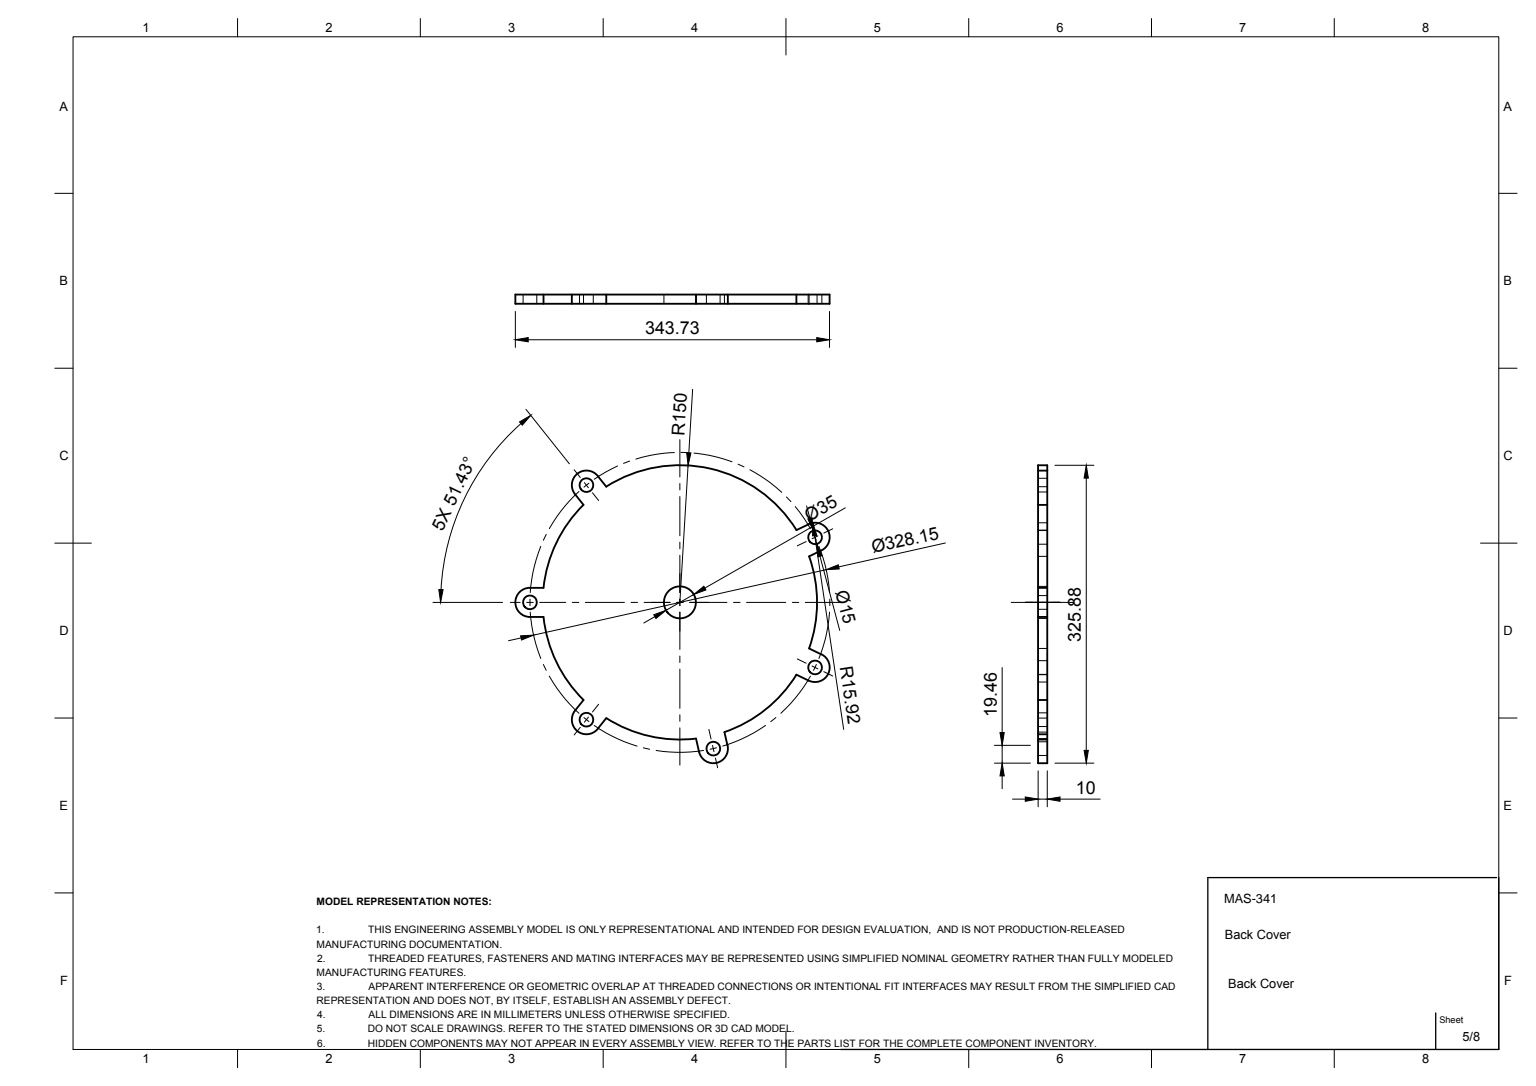
ISO-10303-21;
HEADER;
FILE_DESCRIPTION (('STEP AP214'),
    '1' );
FILE_NAME ('Back Cover.step',
    '2026-10-08T00:39:10',
    ( '' ),
    ( '' ),
    'SwSTEP 2.0',
    'SolidWorks 2025',
    '' );
FILE_SCHEMA (( 'AUTOMOTIVE_DESIGN' ));
ENDSEC;

DATA;
#4=PRODUCT ( 'Back Cover', 'Back Cover', '', ( #531 ) ) ;
#10=VERTEX_POINT ( 'NONE', #9173 ) ;
#12=( GEOMETRIC_REPRESENTATION_CONTEXT ( 3 ) GLOBAL_UNCERTAINTY_ASSIGNED_CONTEXT ( ( #1291 ) ) GLOBAL_UNIT_ASSIGNED_CONTEXT ( ( #18131, #16699, #13613 ) ) REPRESENTATION_CONTEXT ( 'NONE', 'WORKASPACE' ) );
#25=ORIENTED_EDGE ( 'NONE', *, *, #13470, .F. ) ;
#39=DIRECTION ( 'NONE',  ( 0.000000000000000000, 0.000000000000000000, 1.000000000000000000 ) ) ;
#57=CARTESIAN_POINT ( 'NONE',  ( -50.37374754117255549, -141.2886604036510221, 60.00000000000000000 ) ) ;
#62=ORIENTED_EDGE ( 'NONE', *, *, #6982, .T. ) ;
#74=DIRECTION ( 'NONE',  ( -0.000000000000000000, -0.000000000000000000, -1.000000000000000000 ) ) ;
#80=EDGE_LOOP ( 'NONE', ( #725, #12520, #18539, #7460 ) ) ;
#92=CARTESIAN_POINT ( 'NONE',  ( 128.2779226595531270, 102.2982297021113141, 60.00000000000000000 ) ) ;
#95=ORIENTED_EDGE ( 'NONE', *, *, #17125, .F. ) ;
#100=FACE_BOUND ( 'NONE', #8738, .T. ) ;
#107=SURFACE_SIDE_STYLE ('',( #15666 ) ) ;
#135=EDGE_CURVE ( 'NONE', #17975, #14483, #10909, .T. ) ;
#136=CARTESIAN_POINT ( 'NONE',  ( 141.8714406926368099, -48.70825716237082759, 49.99999999999999289 ) ) ;
#173=VECTOR ( 'NONE', #8479, 1000.000000000000000 ) ;
#176=FACE_BOUND ( 'NONE', #16626, .T. ) ;
#187=CYLINDRICAL_SURFACE ( 'NONE', #11980, 150.0000000000000284 ) ;
#205=ORIENTED_EDGE ( 'NONE', *, *, #13470, .T. ) ;
#208=DIRECTION ( 'NONE',  ( 1.000000000000000000, 0.000000000000000000, 0.000000000000000000 ) ) ;
#212=FACE_OUTER_BOUND ( 'NONE', #80, .T. ) ;
#232=DIRECTION ( 'NONE',  ( 1.000000000000000000, 0.000000000000000000, 0.000000000000000000 ) ) ;
#248=CIRCLE ( 'NONE', #6127, 15.91767397667354800 ) ;
#250=ORIENTED_EDGE ( 'NONE', *, *, #6281, .T. ) ;
#254=CARTESIAN_POINT ( 'NONE',  ( 15.91767397667354800, 164.0736214083062805, 49.99999999999999289 ) ) ;
#258=EDGE_CURVE ( 'NONE', #16031, #14304, #11946, .T. ) ;
#262=EDGE_CURVE ( 'NONE', #18721, #13125, #19565, .T. ) ;
#277=FACE_OUTER_BOUND ( 'NONE', #4264, .T. ) ;
#282=DIRECTION ( 'NONE',  ( 4.650550193362991910E-16, 1.000000000000000000, 0.000000000000000000 ) ) ;
#304=FACE_BOUND ( 'NONE', #20117, .T. ) ;
#328=CARTESIAN_POINT ( 'NONE',  ( 85.53020504959901871, -140.9188050298377846, 60.00000000000000000 ) ) ;
#344=VECTOR ( 'NONE', #11455, 1000.000000000000000 ) ;
#372=DIRECTION ( 'NONE',  ( -0.000000000000000000, -0.000000000000000000, -1.000000000000000000 ) ) ;
#377=CARTESIAN_POINT ( 'NONE',  ( 0.000000000000000000, 0.000000000000000000, 49.99999999999999289 ) ) ;
#389=DIRECTION ( 'NONE',  ( -1.000000000000000000, 0.000000000000000000, 0.000000000000000000 ) ) ;
#402=LINE ( 'NONE', #6654, #2889 ) ;
#403=DIRECTION ( 'NONE',  ( 1.000000000000000000, 0.000000000000000000, -0.000000000000000000 ) ) ;
#431=ORIENTED_EDGE ( 'NONE', *, *, #9079, .T. ) ;
#442=DIRECTION ( 'NONE',  ( -0.000000000000000000, -0.000000000000000000, -1.000000000000000000 ) ) ;
#473=VECTOR ( 'NONE', #13912, 1000.000000000000000 ) ;
#531=PRODUCT_CONTEXT ( 'NONE', #16261, 'mechanical' ) ;
#599=VERTEX_POINT ( 'NONE', #13287 ) ;
#600=FACE_OUTER_BOUND ( 'NONE', #14957, .T. ) ;
#615=FACE_OUTER_BOUND ( 'NONE', #9474, .T. ) ;
#625=VERTEX_POINT ( 'NONE', #8798 ) ;
#698=VERTEX_POINT ( 'NONE', #1222 ) ;
#706=ORIENTED_EDGE ( 'NONE', *, *, #12017, .T. ) ;
#711=ORIENTED_EDGE ( 'NONE', *, *, #14248, .F. ) ;
#718=DIRECTION ( 'NONE',  ( -0.9749279121818223981, -0.2225209339563194721, 0.000000000000000000 ) ) ;
#725=ORIENTED_EDGE ( 'NONE', *, *, #984, .T. ) ;
#741=CARTESIAN_POINT ( 'NONE',  ( 141.8714406926368099, -48.70825716237082759, 60.00000000000000000 ) ) ;
#743=CIRCLE ( 'NONE', #20010, 15.91767397667354089 ) ;
#760=CARTESIAN_POINT ( 'NONE',  ( 56.84754764479241373, -154.7316448359447634, 60.00000000000000000 ) ) ;
#773=LINE ( 'NONE', #10087, #5009 ) ;
#778=DIRECTION ( 'NONE',  ( 1.000000000000000000, 0.000000000000000000, 0.000000000000000000 ) ) ;
#798=CARTESIAN_POINT ( 'NONE',  ( 128.2779226595531270, 102.2982297021113141, 60.00000000000000000 ) ) ;
#813=ORIENTED_EDGE ( 'NONE', *, *, #1509, .F. ) ;
#833=AXIS2_PLACEMENT_3D ( 'NONE', #13835, #20185, #6186 ) ;
#847=ADVANCED_FACE ( 'NONE', ( #7869, #100, #5022, #11349, #3578, #17601, #304, #15753 ), #19234, .F. ) ;
#856=DIRECTION ( 'NONE',  ( -1.000000000000000000, 0.000000000000000000, 0.000000000000000000 ) ) ;
#882=DIRECTION ( 'NONE',  ( -0.000000000000000000, -0.000000000000000000, -1.000000000000000000 ) ) ;
#889=EDGE_LOOP ( 'NONE', ( #62, #9459, #3655, #15133 ) ) ;
#893=CIRCLE ( 'NONE', #19539, 15.91767397667354089 ) ;
#900=ORIENTED_EDGE ( 'NONE', *, *, #1584, .T. ) ;
#916=ORIENTED_EDGE ( 'NONE', *, *, #9093, .F. ) ;
#918=ORIENTED_EDGE ( 'NONE', *, *, #10465, .F. ) ;
#922=AXIS2_PLACEMENT_3D ( 'NONE', #2246, #13164, #10012 ) ;
#941=ORIENTED_EDGE ( 'NONE', *, *, #6979, .T. ) ;
#958=ORIENTED_EDGE ( 'NONE', *, *, #5414, .T. ) ;
#984=EDGE_CURVE ( 'NONE', #6115, #9946, #10014, .T. ) ;
#987=EDGE_CURVE ( 'NONE', #11007, #1319, #6991, .T. ) ;
#992=ORIENTED_EDGE ( 'NONE', *, *, #14786, .F. ) ;
#1011=CYLINDRICAL_SURFACE ( 'NONE', #6981, 17.50000000000000355 ) ;
#1018=FACE_OUTER_BOUND ( 'NONE', #6672, .T. ) ;
#1043=DIRECTION ( 'NONE',  ( -0.9749279121818226201, -0.2225209339563185285, 0.000000000000000000 ) ) ;
#1063=DIRECTION ( 'NONE',  ( 1.000000000000000000, 0.000000000000000000, 0.000000000000000000 ) ) ;
#1088=CARTESIAN_POINT ( 'NONE',  ( 71.18887634719571622, -147.8252249328912740, 60.00000000000000000 ) ) ;
#1092=CARTESIAN_POINT ( 'NONE',  ( 148.9554720520395392, -17.67108784863215476, 60.00000000000000000 ) ) ;
#1105=PLANE ( 'NONE',  #9572 ) ;
#1107=CARTESIAN_POINT ( 'NONE',  ( 71.18887634719571622, -147.8252249328912740, 60.00000000000000000 ) ) ;
#1113=( GEOMETRIC_REPRESENTATION_CONTEXT ( 3 ) GLOBAL_UNCERTAINTY_ASSIGNED_CONTEXT ( ( #10482 ) ) GLOBAL_UNIT_ASSIGNED_CONTEXT ( ( #20157, #10630, #1338 ) ) REPRESENTATION_CONTEXT ( 'NONE', 'WORKASPACE' ) );
#1133=ORIENTED_EDGE ( 'NONE', *, *, #5414, .F. ) ;
#1142=DIRECTION ( 'NONE',  ( 1.000000000000000000, 0.000000000000000000, 0.000000000000000000 ) ) ;
#1150=AXIS2_PLACEMENT_3D ( 'NONE', #10589, #13768, #9061 ) ;
#1174=CYLINDRICAL_SURFACE ( 'NONE', #13335, 7.500000000000020428 ) ;
#1181=AXIS2_PLACEMENT_3D ( 'NONE', #18694, #7526, #4675 ) ;
#1195=LINE ( 'NONE', #13780, #11300 ) ;
#1222=CARTESIAN_POINT ( 'NONE',  ( -150.0000000000000284, 0.000000000000000000, 60.00000000000000000 ) ) ;
#1247=AXIS2_PLACEMENT_3D ( 'NONE', #7167, #11750, #11657 ) ;
#1257=CARTESIAN_POINT ( 'NONE',  ( 141.8714406926368099, -48.70825716237082759, 60.00000000000000000 ) ) ;
#1289=DIRECTION ( 'NONE',  ( -0.000000000000000000, -0.000000000000000000, -1.000000000000000000 ) ) ;
#1291=UNCERTAINTY_MEASURE_WITH_UNIT (LENGTH_MEASURE( 1.000000000000000082E-05 ), #18131, 'distance_accuracy_value', 'NONE');
#1305=FACE_BOUND ( 'NONE', #15828, .T. ) ;
#1307=CYLINDRICAL_SURFACE ( 'NONE', #14633, 17.50000000000000355 ) ;
#1319=VERTEX_POINT ( 'NONE', #4241 ) ;
#1326=CARTESIAN_POINT ( 'NONE',  ( 0.000000000000000000, 164.0736214083062805, 60.00000000000000000 ) ) ;
#1338=( NAMED_UNIT ( * ) SI_UNIT ( $, .STERADIAN. ) SOLID_ANGLE_UNIT ( ) );
#1349=AXIS2_PLACEMENT_3D ( 'NONE', #5968, #6073, #13726 ) ;
#1353=VERTEX_POINT ( 'NONE', #2819 ) ;
#1363=LINE ( 'NONE', #10556, #11446 ) ;
#1364=FACE_OUTER_BOUND ( 'NONE', #20043, .T. ) ;
#1380=CARTESIAN_POINT ( 'NONE',  ( 118.3534152657848608, 114.7431683447366595, 60.00000000000000000 ) ) ;
#1381=ORIENTED_EDGE ( 'NONE', *, *, #135, .F. ) ;
#1385=ORIENTED_EDGE ( 'NONE', *, *, #16744, .T. ) ;
#1390=CIRCLE ( 'NONE', #8571, 150.0000000000000284 ) ;
#1400=AXIS2_PLACEMENT_3D ( 'NONE', #17477, #9487, #3450 ) ;
#1418=CIRCLE ( 'NONE', #15461, 150.0000000000000284 ) ;
#1445=DIRECTION ( 'NONE',  ( -0.000000000000000000, -0.000000000000000000, -1.000000000000000000 ) ) ;
#1472=EDGE_CURVE ( 'NONE', #8799, #13849, #8940, .T. ) ;
#1509=EDGE_CURVE ( 'NONE', #4476, #12253, #6504, .T. ) ;
#1519=LINE ( 'NONE', #7852, #19488 ) ;
#1524=CARTESIAN_POINT ( 'NONE',  ( 17.50000000000001776, 2.143131898507868643E-15, 60.00000000000000000 ) ) ;
#1529=AXIS2_PLACEMENT_3D ( 'NONE', #19924, #15537, #18818 ) ;
#1552=AXIS2_PLACEMENT_3D ( 'NONE', #4912, #17489, #14204 ) ;
#1579=AXIS2_PLACEMENT_3D ( 'NONE', #1380, #7217, #12522 ) ;
#1581=ORIENTED_EDGE ( 'NONE', *, *, #6806, .T. ) ;
#1584=EDGE_CURVE ( 'NONE', #11084, #12677, #9359, .T. ) ;
#1604=EDGE_LOOP ( 'NONE', ( #11796, #250, #431, #18706 ) ) ;
#1610=ORIENTED_EDGE ( 'NONE', *, *, #6423, .F. ) ;
#1617=DIRECTION ( 'NONE',  ( 1.000000000000000000, 0.000000000000000000, -0.000000000000000000 ) ) ;
#1632=CARTESIAN_POINT ( 'NONE',  ( 85.53020504959901871, -140.9188050298377846, 60.00000000000000000 ) ) ;
#1641=DIRECTION ( 'NONE',  ( -0.000000000000000000, -0.000000000000000000, -1.000000000000000000 ) ) ;
#1643=ADVANCED_BREP_SHAPE_REPRESENTATION ( '', ( #14854, #18639 ), #12 ) ;
#1668=ORIENTED_EDGE ( 'NONE', *, *, #10953, .T. ) ;
#1674=LINE ( 'NONE', #5228, #9676 ) ;
#1681=VERTEX_POINT ( 'NONE', #19287 ) ;
#1690=CARTESIAN_POINT ( 'NONE',  ( -152.4599531637108498, -36.50981547337168109, 60.00000000000000000 ) ) ;
#1697=DIRECTION ( 'NONE',  ( 1.000000000000000000, 0.000000000000000000, 0.000000000000000000 ) ) ;
#1711=CARTESIAN_POINT ( 'NONE',  ( 0.000000000000000000, 164.0736214083062805, 49.99999999999999289 ) ) ;
#1735=ORIENTED_EDGE ( 'NONE', *, *, #7341, .T. ) ;
#1740=EDGE_CURVE ( 'NONE', #6676, #16987, #17142, .T. ) ;
#1778=DIRECTION ( 'NONE',  ( 0.000000000000000000, 0.000000000000000000, 1.000000000000000000 ) ) ;
#1782=ADVANCED_FACE ( 'NONE', ( #12080 ), #4425, .T. ) ;
#1806=EDGE_LOOP ( 'NONE', ( #13482, #12155, #3837, #11415 ) ) ;
#1818=DIRECTION ( 'NONE',  ( 1.000000000000000000, -4.650550193362991910E-16, 0.000000000000000000 ) ) ;
#1822=CARTESIAN_POINT ( 'NONE',  ( -156.4179374840092862, -52.02840013024096066, 49.99999999999999289 ) ) ;
#1828=CIRCLE ( 'NONE', #15542, 7.500000000000007105 ) ;
#1843=LINE ( 'NONE', #8280, #16385 ) ;
#1850=EDGE_CURVE ( 'NONE', #9217, #15200, #9187, .T. ) ;
#1873=CYLINDRICAL_SURFACE ( 'NONE', #16470, 15.91767397667354089 ) ;
#1887=VERTEX_POINT ( 'NONE', #4317 ) ;
#1888=CIRCLE ( 'NONE', #17570, 15.91767397667354089 ) ;
#1890=EDGE_LOOP ( 'NONE', ( #916, #3438, #11512, #2174 ) ) ;
#1897=LINE ( 'NONE', #11196, #7566 ) ;
#1903=EDGE_CURVE ( 'NONE', #17877, #8041, #1843, .T. ) ;
#1907=EDGE_CURVE ( 'NONE', #16556, #4476, #3003, .T. ) ;
#1926=LINE ( 'NONE', #17482, #13030 ) ;
#1998=PLANE ( 'NONE',  #3865 ) ;
#2007=CIRCLE ( 'NONE', #16700, 7.500000000000008882 ) ;
#2015=ADVANCED_FACE ( 'NONE', ( #9948 ), #13293, .T. ) ;
#2032=CARTESIAN_POINT ( 'NONE',  ( 152.4599531637113330, -36.50981547336952104, 60.00000000000000000 ) ) ;
#2035=CARTESIAN_POINT ( 'NONE',  ( 152.4599531637113330, -36.50981547336952104, 60.00000000000000000 ) ) ;
#2037=CYLINDRICAL_SURFACE ( 'NONE', #2496, 7.500000000000008882 ) ;
#2058=DIRECTION ( 'NONE',  ( 1.000000000000000000, 0.000000000000000000, 0.000000000000000000 ) ) ;
#2066=EDGE_LOOP ( 'NONE', ( #20041, #7947, #14391, #7069 ) ) ;
#2073=VECTOR ( 'NONE', #9324, 1000.000000000000114 ) ;
#2075=ORIENTED_EDGE ( 'NONE', *, *, #3500, .F. ) ;
#2082=ORIENTED_EDGE ( 'NONE', *, *, #2486, .T. ) ;
#2109=VERTEX_POINT ( 'NONE', #15142 ) ;
#2110=ORIENTED_EDGE ( 'NONE', *, *, #18540, .T. ) ;
#2133=CYLINDRICAL_SURFACE ( 'NONE', #18006, 7.500000000000007105 ) ;
#2140=LINE ( 'NONE', #17790, #20045 ) ;
#2143=VECTOR ( 'NONE', #3874, 1000.000000000000000 ) ;
#2168=DIRECTION ( 'NONE',  ( -1.000000000000000000, 0.000000000000000000, 0.000000000000000000 ) ) ;
#2172=ADVANCED_FACE ( 'NONE', ( #8056 ), #2133, .F. ) ;
#2174=ORIENTED_EDGE ( 'NONE', *, *, #10355, .F. ) ;
#2177=ADVANCED_FACE ( 'NONE', ( #16047 ), #13058, .F. ) ;
#2206=CARTESIAN_POINT ( 'NONE',  ( -71.18887634719365565, -147.8252249328922687, 60.00000000000000000 ) ) ;
#2240=ORIENTED_EDGE ( 'NONE', *, *, #12488, .F. ) ;
#2245=ORIENTED_EDGE ( 'NONE', *, *, #15519, .T. ) ;
#2246=CARTESIAN_POINT ( 'NONE',  ( 126.5370453525553671, 80.55045718954892209, 60.00000000000000000 ) ) ;
#2257=CARTESIAN_POINT ( 'NONE',  ( 0.000000000000000000, 0.000000000000000000, 49.99999999999999289 ) ) ;
#2269=VERTEX_POINT ( 'NONE', #8950 ) ;
#2273=VECTOR ( 'NONE', #9693, 1000.000000000000000 ) ;
#2302=ADVANCED_FACE ( 'NONE', ( #11913 ), #19800, .T. ) ;
#2330=CARTESIAN_POINT ( 'NONE',  ( -148.9554720520392834, -17.67108784863415138, 60.00000000000000000 ) ) ;
#2335=ORIENTED_EDGE ( 'NONE', *, *, #16292, .F. ) ;
#2359=CARTESIAN_POINT ( 'NONE',  ( 128.2779226595531270, 102.2982297021113141, 49.99999999999999289 ) ) ;
#2362=VERTEX_POINT ( 'NONE', #16735 ) ;
#2367=VECTOR ( 'NONE', #7281, 1000.000000000000000 ) ;
#2405=DIRECTION ( 'NONE',  ( -0.000000000000000000, -0.000000000000000000, -1.000000000000000000 ) ) ;
#2422=ORIENTED_EDGE ( 'NONE', *, *, #19415, .T. ) ;
#2429=CARTESIAN_POINT ( 'NONE',  ( -175.8776271403844191, -36.50981547337168109, 60.00000000000000000 ) ) ;
#2445=DIRECTION ( 'NONE',  ( -0.000000000000000000, -0.000000000000000000, -1.000000000000000000 ) ) ;
#2486=EDGE_CURVE ( 'NONE', #1353, #1681, #14082, .T. ) ;
#2496=AXIS2_PLACEMENT_3D ( 'NONE', #11129, #17390, #3567 ) ;
#2525=EDGE_CURVE ( 'NONE', #10243, #10598, #19835, .T. ) ;
#2540=CIRCLE ( 'NONE', #3850, 150.0000000000000284 ) ;
#2550=CARTESIAN_POINT ( 'NONE',  ( -63.68887634719364144, -147.8252249328922687, 49.99999999999999289 ) ) ;
#2553=AXIS2_PLACEMENT_3D ( 'NONE', #8742, #16438, #11428 ) ;
#2606=CARTESIAN_POINT ( 'NONE',  ( 118.3534152657848608, 114.7431683447366595, 60.00000000000000000 ) ) ;
#2630=EDGE_CURVE ( 'NONE', #7170, #17394, #19295, .T. ) ;
#2660=FACE_OUTER_BOUND ( 'NONE', #2066, .T. ) ;
#2663=EDGE_LOOP ( 'NONE', ( #8353, #3788, #6370, #3707 ) ) ;
#2673=EDGE_CURVE ( 'NONE', #19329, #4234, #19485, .T. ) ;
#2680=ORIENTED_EDGE ( 'NONE', *, *, #4734, .T. ) ;
#2702=DIRECTION ( 'NONE',  ( -0.000000000000000000, -0.000000000000000000, -1.000000000000000000 ) ) ;
#2720=VERTEX_POINT ( 'NONE', #5377 ) ;
#2762=FACE_OUTER_BOUND ( 'NONE', #5149, .T. ) ;
#2769=ADVANCED_FACE ( 'NONE', ( #4030 ), #3930, .F. ) ;
#2771=EDGE_LOOP ( 'NONE', ( #13142, #16829 ) ) ;
#2799=DIRECTION ( 'NONE',  ( -0.000000000000000000, -0.000000000000000000, -1.000000000000000000 ) ) ;
#2819=CARTESIAN_POINT ( 'NONE',  ( 78.68887634719573043, -147.8252249328912740, 49.99999999999999289 ) ) ;
#2822=DIRECTION ( 'NONE',  ( 0.000000000000000000, 0.000000000000000000, 1.000000000000000000 ) ) ;
#2861=CARTESIAN_POINT ( 'NONE',  ( 159.9599531637113330, -36.50981547336952104, 49.99999999999999289 ) ) ;
#2874=ADVANCED_FACE ( 'NONE', ( #19877 ), #13943, .F. ) ;
#2889=VECTOR ( 'NONE', #11447, 1000.000000000000000 ) ;
#2909=CIRCLE ( 'NONE', #10735, 7.500000000000007105 ) ;
#2931=APPLICATION_CONTEXT ( 'automotive_design' ) ;
#2936=VECTOR ( 'NONE', #1641, 1000.000000000000000 ) ;
#2941=ORIENTED_EDGE ( 'NONE', *, *, #2525, .T. ) ;
#2965=ORIENTED_EDGE ( 'NONE', *, *, #17308, .F. ) ;
#2967=ORIENTED_EDGE ( 'NONE', *, *, #5286, .T. ) ;
#2975=EDGE_CURVE ( 'NONE', #16978, #16987, #10665, .T. ) ;
#2986=ORIENTED_EDGE ( 'NONE', *, *, #19843, .F. ) ;
#2988=CARTESIAN_POINT ( 'NONE',  ( -156.4179374840092862, -52.02840013024096066, 49.99999999999999289 ) ) ;
#3003=LINE ( 'NONE', #19237, #3320 ) ;
#3015=CIRCLE ( 'NONE', #18700, 7.500000000000007105 ) ;
#3025=PLANE ( 'NONE',  #1579 ) ;
#3101=LINE ( 'NONE', #15578, #9580 ) ;
#3124=DIRECTION ( 'NONE',  ( -0.000000000000000000, -0.000000000000000000, -1.000000000000000000 ) ) ;
#3135=DIRECTION ( 'NONE',  ( 1.000000000000000000, 0.000000000000000000, 0.000000000000000000 ) ) ;
#3146=AXIS2_PLACEMENT_3D ( 'NONE', #17379, #3352, #9591 ) ;
#3160=EDGE_LOOP ( 'NONE', ( #19301, #4729, #13376, #19732 ) ) ;
#3192=DIRECTION ( 'NONE',  ( 0.000000000000000000, 0.000000000000000000, 1.000000000000000000 ) ) ;
#3195=ORIENTED_EDGE ( 'NONE', *, *, #8308, .T. ) ;
#3223=VECTOR ( 'NONE', #74, 1000.000000000000000 ) ;
#3229=ADVANCED_FACE ( 'NONE', ( #16398 ), #15050, .T. ) ;
#3231=CARTESIAN_POINT ( 'NONE',  ( 120.7779226595530986, 102.2982297021113141, 60.00000000000000000 ) ) ;
#3233=DIRECTION ( 'NONE',  ( 0.000000000000000000, 0.000000000000000000, 1.000000000000000000 ) ) ;
#3243=ADVANCED_FACE ( 'NONE', ( #7276 ), #7083, .T. ) ;
#3264=DIRECTION ( 'NONE',  ( -0.000000000000000000, -0.000000000000000000, -1.000000000000000000 ) ) ;
#3267=FACE_OUTER_BOUND ( 'NONE', #1604, .T. ) ;
#3275=PRODUCT_DEFINITION ( 'UNKNOWN', '', #10143, #7010 ) ;
#3308=CIRCLE ( 'NONE', #19312, 150.0000000000000284 ) ;
#3316=CARTESIAN_POINT ( 'NONE',  ( 159.9599531637113330, -36.50981547336952104, 60.00000000000000000 ) ) ;
#3320=VECTOR ( 'NONE', #3679, 1000.000000000000000 ) ;
#3327=DIRECTION ( 'NONE',  ( -0.7818314824680222541, -0.6234898018587428092, 0.000000000000000000 ) ) ;
#3330=CARTESIAN_POINT ( 'NONE',  ( 71.18887634719571622, -147.8252249328912740, 60.00000000000000000 ) ) ;
#3341=EDGE_LOOP ( 'NONE', ( #9492, #4784, #5801, #2110, #12859, #14208, #1735, #19633, #12646, #958, #17042, #11082, #11220, #15387, #15418, #2422, #7191, #11685, #1581, #3959, #19178, #18458, #2245, #18129, #7799, #17297, #2967 ) ) ;
#3352=DIRECTION ( 'NONE',  ( 0.000000000000000000, 0.000000000000000000, 1.000000000000000000 ) ) ;
#3391=DIRECTION ( 'NONE',  ( 0.000000000000000000, 0.000000000000000000, 1.000000000000000000 ) ) ;
#3401=EDGE_CURVE ( 'NONE', #17191, #3695, #12037, .T. ) ;
#3407=VECTOR ( 'NONE', #8574, 1000.000000000000000 ) ;
#3438=ORIENTED_EDGE ( 'NONE', *, *, #3401, .T. ) ;
#3450=DIRECTION ( 'NONE',  ( -0.4338837391175549008, -0.9009688679024205893, 0.000000000000000000 ) ) ;
#3452=DIRECTION ( 'NONE',  ( 0.000000000000000000, 0.000000000000000000, 1.000000000000000000 ) ) ;
#3453=EDGE_LOOP ( 'NONE', ( #11712, #4339, #4209, #20136 ) ) ;
#3457=CARTESIAN_POINT ( 'NONE',  ( 0.000000000000000000, 164.0736214083062805, 60.00000000000000000 ) ) ;
#3458=LINE ( 'NONE', #2032, #2273 ) ;
#3490=AXIS2_PLACEMENT_3D ( 'NONE', #3457, #15736, #19021 ) ;
#3491=ORIENTED_EDGE ( 'NONE', *, *, #17032, .T. ) ;
#3493=DIRECTION ( 'NONE',  ( -1.000000000000000000, 4.650550193362991910E-16, 0.000000000000000000 ) ) ;
#3494=CARTESIAN_POINT ( 'NONE',  ( 50.37374754117451658, -141.2886604036503115, 49.99999999999999289 ) ) ;
#3500=EDGE_CURVE ( 'NONE', #4491, #18721, #7194, .T. ) ;
#3515=DIRECTION ( 'NONE',  ( 0.4338837391175662250, -0.9009688679024151492, 0.000000000000000000 ) ) ;
#3558=FACE_OUTER_BOUND ( 'NONE', #9060, .T. ) ;
#3567=DIRECTION ( 'NONE',  ( -1.000000000000000000, 0.000000000000000000, 0.000000000000000000 ) ) ;
#3568=VECTOR ( 'NONE', #3852, 1000.000000000000227 ) ;
#3569=CIRCLE ( 'NONE', #3896, 150.0000000000000284 ) ;
#3577=PLANE ( 'NONE',  #922 ) ;
#3578=FACE_BOUND ( 'NONE', #16226, .T. ) ;
#3595=DIRECTION ( 'NONE',  ( -4.650550193362991910E-16, -1.000000000000000000, 0.000000000000000000 ) ) ;
#3601=ORIENTED_EDGE ( 'NONE', *, *, #6285, .T. ) ;
#3606=CARTESIAN_POINT ( 'NONE',  ( -85.53020504959707182, -140.9188050298390067, 49.99999999999999289 ) ) ;
#3617=FACE_OUTER_BOUND ( 'NONE', #19792, .T. ) ;
#3620=VERTEX_POINT ( 'NONE', #14922 ) ;
#3639=AXIS2_PLACEMENT_3D ( 'NONE', #5062, #11284, #4960 ) ;
#3642=EDGE_LOOP ( 'NONE', ( #9938, #13927 ) ) ;
#3655=ORIENTED_EDGE ( 'NONE', *, *, #17655, .F. ) ;
#3672=ORIENTED_EDGE ( 'NONE', *, *, #18599, .F. ) ;
#3674=DIRECTION ( 'NONE',  ( 1.000000000000000000, 0.000000000000000000, 0.000000000000000000 ) ) ;
#3679=DIRECTION ( 'NONE',  ( -0.000000000000000000, -0.000000000000000000, -1.000000000000000000 ) ) ;
#3695=VERTEX_POINT ( 'NONE', #16669 ) ;
#3699=CIRCLE ( 'NONE', #14151, 7.500000000000020428 ) ;
#3700=VERTEX_POINT ( 'NONE', #15326 ) ;
#3702=ORIENTED_EDGE ( 'NONE', *, *, #4419, .T. ) ;
#3707=ORIENTED_EDGE ( 'NONE', *, *, #6423, .T. ) ;
#3723=DIRECTION ( 'NONE',  ( 0.000000000000000000, 0.000000000000000000, 1.000000000000000000 ) ) ;
#3732=DIRECTION ( 'NONE',  ( 0.7818314824680226982, 0.6234898018587423651, 0.000000000000000000 ) ) ;
#3738=COLOUR_RGB ( '', 0.66274510, 0.83137255, 0.94901961) ;
#3756=CARTESIAN_POINT ( 'NONE',  ( -167.4599531637108782, -36.50981547337168109, 60.00000000000000000 ) ) ;
#3760=DIRECTION ( 'NONE',  ( -0.000000000000000000, -0.000000000000000000, -1.000000000000000000 ) ) ;
#3764=CARTESIAN_POINT ( 'NONE',  ( -50.37374754117255549, -141.2886604036510221, 60.00000000000000000 ) ) ;
#3788=ORIENTED_EDGE ( 'NONE', *, *, #19393, .F. ) ;
#3797=ORIENTED_EDGE ( 'NONE', *, *, #4544, .F. ) ;
#3837=ORIENTED_EDGE ( 'NONE', *, *, #10862, .T. ) ;
#3850=AXIS2_PLACEMENT_3D ( 'NONE', #12740, #19000, #17466 ) ;
#3852=DIRECTION ( 'NONE',  ( -0.9749279121818223981, -0.2225209339563194721, 0.000000000000000000 ) ) ;
#3855=EDGE_CURVE ( 'NONE', #4788, #2109, #15644, .T. ) ;
#3858=CARTESIAN_POINT ( 'NONE',  ( 135.7779226595531270, 102.2982297021113141, 49.99999999999999289 ) ) ;
#3859=LINE ( 'NONE', #8464, #5451 ) ;
#3865=AXIS2_PLACEMENT_3D ( 'NONE', #18551, #4426, #1043 ) ;
#3869=ORIENTED_EDGE ( 'NONE', *, *, #5675, .F. ) ;
#3874=DIRECTION ( 'NONE',  ( -0.000000000000000000, -0.000000000000000000, -1.000000000000000000 ) ) ;
#3880=CARTESIAN_POINT ( 'NONE',  ( -79.05640494597940915, -127.4758205975444270, 60.00000000000000000 ) ) ;
#3896=AXIS2_PLACEMENT_3D ( 'NONE', #11016, #14092, #15733 ) ;
#3897=EDGE_CURVE ( 'NONE', #16737, #6676, #19883, .T. ) ;
#3906=CARTESIAN_POINT ( 'NONE',  ( 50.37374754117451658, -141.2886604036503115, 60.00000000000000000 ) ) ;
#3911=ORIENTED_EDGE ( 'NONE', *, *, #5282, .T. ) ;
#3930=PLANE ( 'NONE',  #4819 ) ;
#3934=VERTEX_POINT ( 'NONE', #19222 ) ;
#3938=VERTEX_POINT ( 'NONE', #3858 ) ;
#3949=LINE ( 'NONE', #16446, #13934 ) ;
#3959=ORIENTED_EDGE ( 'NONE', *, *, #5121, .T. ) ;
#3967=FACE_OUTER_BOUND ( 'NONE', #15282, .T. ) ;
#3973=DIRECTION ( 'NONE',  ( 1.000000000000000000, 0.000000000000000000, 0.000000000000000000 ) ) ;
#3983=ORIENTED_EDGE ( 'NONE', *, *, #12666, .T. ) ;
#3996=AXIS2_PLACEMENT_3D ( 'NONE', #19556, #11767, #8709 ) ;
#4014=ORIENTED_EDGE ( 'NONE', *, *, #17032, .F. ) ;
#4030=FACE_OUTER_BOUND ( 'NONE', #13227, .T. ) ;
#4056=ORIENTED_EDGE ( 'NONE', *, *, #17125, .T. ) ;
#4064=DIRECTION ( 'NONE',  ( 1.000000000000000000, 0.000000000000000000, 0.000000000000000000 ) ) ;
#4069=ORIENTED_EDGE ( 'NONE', *, *, #5286, .F. ) ;
#4071=DIRECTION ( 'NONE',  ( 0.000000000000000000, 0.000000000000000000, 1.000000000000000000 ) ) ;
#4082=DIRECTION ( 'NONE',  ( 0.000000000000000000, 0.000000000000000000, 1.000000000000000000 ) ) ;
#4092=DIRECTION ( 'NONE',  ( -0.000000000000000000, -0.000000000000000000, -1.000000000000000000 ) ) ;
#4098=DIRECTION ( 'NONE',  ( 1.000000000000000000, 0.000000000000000000, 0.000000000000000000 ) ) ;
#4122=ORIENTED_EDGE ( 'NONE', *, *, #5532, .T. ) ;
#4129=DIRECTION ( 'NONE',  ( 0.000000000000000000, 0.000000000000000000, 1.000000000000000000 ) ) ;
#4166=VECTOR ( 'NONE', #10347, 1000.000000000000000 ) ;
#4183=AXIS2_PLACEMENT_3D ( 'NONE', #16892, #9107, #208 ) ;
#4191=CARTESIAN_POINT ( 'NONE',  ( -79.05640494597940915, -127.4758205975444270, 49.99999999999999289 ) ) ;
#4203=CYLINDRICAL_SURFACE ( 'NONE', #18192, 150.0000000000000284 ) ;
#4209=ORIENTED_EDGE ( 'NONE', *, *, #11907, .F. ) ;
#4234=VERTEX_POINT ( 'NONE', #9956 ) ;
#4235=CARTESIAN_POINT ( 'NONE',  ( -78.68887634719368407, -147.8252249328922687, 60.00000000000000000 ) ) ;
#4241=CARTESIAN_POINT ( 'NONE',  ( 135.7779226595531270, 102.2982297021113141, 60.00000000000000000 ) ) ;
#4247=EDGE_CURVE ( 'NONE', #1319, #3938, #19560, .T. ) ;
#4264=EDGE_LOOP ( 'NONE', ( #4368, #6719, #5070, #9063 ) ) ;
#4274=ORIENTED_EDGE ( 'NONE', *, *, #11719, .T. ) ;
#4283=CIRCLE ( 'NONE', #14745, 7.500000000000020428 ) ;
#4300=PRESENTATION_STYLE_ASSIGNMENT (( #7468 ) ) ;
#4317=CARTESIAN_POINT ( 'NONE',  ( -79.05640494597940915, -127.4758205975444270, 60.00000000000000000 ) ) ;
#4328=DIRECTION ( 'NONE',  ( 0.4338837391175509040, 0.9009688679024224767, 0.000000000000000000 ) ) ;
#4339=ORIENTED_EDGE ( 'NONE', *, *, #3855, .F. ) ;
#4367=ORIENTED_EDGE ( 'NONE', *, *, #1903, .T. ) ;
#4368=ORIENTED_EDGE ( 'NONE', *, *, #12488, .T. ) ;
#4371=CARTESIAN_POINT ( 'NONE',  ( 106.6880305650188347, 105.4403344747995988, 49.99999999999999289 ) ) ;
#4373=DIRECTION ( 'NONE',  ( 4.650550193362991910E-16, 1.000000000000000000, 0.000000000000000000 ) ) ;
#4374=CARTESIAN_POINT ( 'NONE',  ( -141.8714406926361562, -48.70825716237266079, 49.99999999999999289 ) ) ;
#4395=ORIENTED_EDGE ( 'NONE', *, *, #6979, .F. ) ;
#4419=EDGE_CURVE ( 'NONE', #18721, #17815, #6063, .T. ) ;
#4425=CYLINDRICAL_SURFACE ( 'NONE', #10923, 150.0000000000000284 ) ;
#4426=DIRECTION ( 'NONE',  ( -0.2225209339563185562, 0.9749279121818227312, 0.000000000000000000 ) ) ;
#4431=DIRECTION ( 'NONE',  ( -0.9749279121818255067, 0.2225209339563057331, 0.000000000000000000 ) ) ;
#4444=AXIS2_PLACEMENT_3D ( 'NONE', #10484, #15616, #18279 ) ;
#4463=CARTESIAN_POINT ( 'NONE',  ( -15.91767397667354800, 164.0736214083062805, 60.00000000000000000 ) ) ;
#4470=FACE_BOUND ( 'NONE', #2771, .T. ) ;
#4476=VERTEX_POINT ( 'NONE', #9008 ) ;
#4490=CYLINDRICAL_SURFACE ( 'NONE', #5988, 7.500000000000007105 ) ;
#4491=VERTEX_POINT ( 'NONE', #4622 ) ;
#4515=LINE ( 'NONE', #5853, #2073 ) ;
#4523=CIRCLE ( 'NONE', #17944, 17.50000000000000355 ) ;
#4544=EDGE_CURVE ( 'NONE', #1887, #17975, #4515, .T. ) ;
#4597=ORIENTED_EDGE ( 'NONE', *, *, #15010, .T. ) ;
#4606=ORIENTED_EDGE ( 'NONE', *, *, #1907, .T. ) ;
#4610=AXIS2_PLACEMENT_3D ( 'NONE', #3316, #11075, #19076 ) ;
#4615=LINE ( 'NONE', #9717, #8243 ) ;
#4619=EDGE_LOOP ( 'NONE', ( #19256, #12856, #8644, #12571 ) ) ;
#4622=CARTESIAN_POINT ( 'NONE',  ( -175.8776271403844191, -36.50981547337168109, 60.00000000000000000 ) ) ;
#4629=VERTEX_POINT ( 'NONE', #3494 ) ;
#4646=DIRECTION ( 'NONE',  ( 0.9009688679024225877, -0.4338837391175509595, 0.000000000000000000 ) ) ;
#4659=CARTESIAN_POINT ( 'NONE',  ( 118.3534152657848608, 114.7431683447366595, 49.99999999999999289 ) ) ;
#4666=ORIENTED_EDGE ( 'NONE', *, *, #6197, .F. ) ;
#4675=DIRECTION ( 'NONE',  ( 1.000000000000000000, 0.000000000000000000, 0.000000000000000000 ) ) ;
#4692=DIRECTION ( 'NONE',  ( -0.9009688679024161484, -0.4338837391175643932, 0.000000000000000000 ) ) ;
#4729=ORIENTED_EDGE ( 'NONE', *, *, #7736, .F. ) ;
#4733=ORIENTED_EDGE ( 'NONE', *, *, #18231, .T. ) ;
#4734=EDGE_CURVE ( 'NONE', #8237, #4476, #743, .T. ) ;
#4739=AXIS2_PLACEMENT_3D ( 'NONE', #18707, #4692, #10915 ) ;
#4744=AXIS2_PLACEMENT_3D ( 'NONE', #9033, #4129, #16145 ) ;
#4749=ADVANCED_FACE ( 'NONE', ( #19636 ), #1011, .F. ) ;
#4776=ADVANCED_FACE ( 'NONE', ( #2762 ), #4490, .F. ) ;
#4777=ORIENTED_EDGE ( 'NONE', *, *, #4870, .F. ) ;
#4784=ORIENTED_EDGE ( 'NONE', *, *, #9415, .T. ) ;
#4788=VERTEX_POINT ( 'NONE', #15437 ) ;
#4811=EDGE_LOOP ( 'NONE', ( #16003, #8956, #15930, #10927 ) ) ;
#4819=AXIS2_PLACEMENT_3D ( 'NONE', #10172, #16521, #14872 ) ;
#4827=DIRECTION ( 'NONE',  ( -0.000000000000000000, -0.000000000000000000, -1.000000000000000000 ) ) ;
#4855=CARTESIAN_POINT ( 'NONE',  ( 0.000000000000000000, 164.0736214083062805, 60.00000000000000000 ) ) ;
#4870=EDGE_CURVE ( 'NONE', #5317, #13849, #11547, .T. ) ;
#4877=DIRECTION ( 'NONE',  ( -1.000000000000000000, 0.000000000000000000, 0.000000000000000000 ) ) ;
#4888=ORIENTED_EDGE ( 'NONE', *, *, #19843, .T. ) ;
#4901=DIRECTION ( 'NONE',  ( 1.000000000000000000, 0.000000000000000000, 0.000000000000000000 ) ) ;
#4912=CARTESIAN_POINT ( 'NONE',  ( 159.9599531637113330, -36.50981547336952104, 60.00000000000000000 ) ) ;
#4926=CARTESIAN_POINT ( 'NONE',  ( 0.000000000000000000, 0.000000000000000000, 49.99999999999999289 ) ) ;
#4934=ORIENTED_EDGE ( 'NONE', *, *, #10382, .F. ) ;
#4940=EDGE_LOOP ( 'NONE', ( #18354, #4934, #19786, #15681 ) ) ;
#4955=ADVANCED_FACE ( 'NONE', ( #10928 ), #18826, .F. ) ;
#4960=DIRECTION ( 'NONE',  ( 1.000000000000000000, 0.000000000000000000, 0.000000000000000000 ) ) ;
#4964=AXIS2_PLACEMENT_3D ( 'NONE', #6977, #16300, #13196 ) ;
#4980=ORIENTED_EDGE ( 'NONE', *, *, #9415, .F. ) ;
#5000=DIRECTION ( 'NONE',  ( -0.000000000000000000, -0.000000000000000000, -1.000000000000000000 ) ) ;
#5005=DIRECTION ( 'NONE',  ( -1.000000000000000000, 0.000000000000000000, 0.000000000000000000 ) ) ;
#5008=VECTOR ( 'NONE', #18332, 1000.000000000000000 ) ;
#5009=VECTOR ( 'NONE', #19865, 1000.000000000000000 ) ;
#5015=DIRECTION ( 'NONE',  ( -1.000000000000000000, 0.000000000000000000, 0.000000000000000000 ) ) ;
#5022=FACE_BOUND ( 'NONE', #13984, .T. ) ;
#5025=VECTOR ( 'NONE', #15688, 1000.000000000000227 ) ;
#5030=DIRECTION ( 'NONE',  ( 0.000000000000000000, 0.000000000000000000, 1.000000000000000000 ) ) ;
#5062=CARTESIAN_POINT ( 'NONE',  ( -159.9599531637108782, -36.50981547337168109, 60.00000000000000000 ) ) ;
#5065=ORIENTED_EDGE ( 'NONE', *, *, #135, .T. ) ;
#5070=ORIENTED_EDGE ( 'NONE', *, *, #13129, .F. ) ;
#5083=VERTEX_POINT ( 'NONE', #19425 ) ;
#5121=EDGE_CURVE ( 'NONE', #10879, #7170, #1418, .T. ) ;
#5149=EDGE_LOOP ( 'NONE', ( #19102, #15112, #4777, #11521 ) ) ;
#5163=DIRECTION ( 'NONE',  ( -0.000000000000000000, -0.000000000000000000, -1.000000000000000000 ) ) ;
#5181=DIRECTION ( 'NONE',  ( -0.9749279121818255067, 0.2225209339563057331, 0.000000000000000000 ) ) ;
#5196=DIRECTION ( 'NONE',  ( 1.000000000000000000, 0.000000000000000000, 0.000000000000000000 ) ) ;
#5197=CIRCLE ( 'NONE', #14001, 15.91767397667354089 ) ;
#5203=ORIENTED_EDGE ( 'NONE', *, *, #18109, .F. ) ;
#5204=DIRECTION ( 'NONE',  ( 0.2225209339563194721, -0.9749279121818225091, 0.000000000000000000 ) ) ;
#5209=DIRECTION ( 'NONE',  ( -0.000000000000000000, -0.000000000000000000, -1.000000000000000000 ) ) ;
#5223=CARTESIAN_POINT ( 'NONE',  ( 17.50000000000001776, 2.143131898507868643E-15, 60.00000000000000000 ) ) ;
#5228=CARTESIAN_POINT ( 'NONE',  ( -15.91767397667354800, 164.0736214083062805, 60.00000000000000000 ) ) ;
#5251=EDGE_CURVE ( 'NONE', #12873, #10598, #2140, .T. ) ;
#5281=EDGE_LOOP ( 'NONE', ( #14805, #992, #6577, #17055 ) ) ;
#5282=EDGE_CURVE ( 'NONE', #5083, #3700, #7694, .T. ) ;
#5286=EDGE_CURVE ( 'NONE', #3620, #16612, #8955, .T. ) ;
#5288=ORIENTED_EDGE ( 'NONE', *, *, #9531, .F. ) ;
#5300=DIRECTION ( 'NONE',  ( 1.000000000000000000, 0.000000000000000000, 0.000000000000000000 ) ) ;
#5316=CARTESIAN_POINT ( 'NONE',  ( -7.500000000000008882, 164.0736214083062805, 60.00000000000000000 ) ) ;
#5317=VERTEX_POINT ( 'NONE', #10695 ) ;
#5323=DIRECTION ( 'NONE',  ( -0.000000000000000000, -0.000000000000000000, -1.000000000000000000 ) ) ;
#5377=CARTESIAN_POINT ( 'NONE',  ( -56.84754764479025368, -154.7316448359455308, 60.00000000000000000 ) ) ;
#5382=CIRCLE ( 'NONE', #7322, 15.91767397667354089 ) ;
#5391=AXIS2_PLACEMENT_3D ( 'NONE', #19017, #1818, #282 ) ;
#5400=DIRECTION ( 'NONE',  ( -0.000000000000000000, -0.000000000000000000, -1.000000000000000000 ) ) ;
#5406=DIRECTION ( 'NONE',  ( 0.000000000000000000, 0.000000000000000000, 1.000000000000000000 ) ) ;
#5408=ORIENTED_EDGE ( 'NONE', *, *, #10832, .F. ) ;
#5414=EDGE_CURVE ( 'NONE', #6230, #2720, #5749, .T. ) ;
#5416=LINE ( 'NONE', #5223, #2143 ) ;
#5425=ORIENTED_EDGE ( 'NONE', *, *, #12017, .F. ) ;
#5446=DIRECTION ( 'NONE',  ( -0.000000000000000000, -0.000000000000000000, -1.000000000000000000 ) ) ;
#5451=VECTOR ( 'NONE', #882, 1000.000000000000000 ) ;
#5452=CARTESIAN_POINT ( 'NONE',  ( 126.5370453525553671, 80.55045718954892209, 49.99999999999999289 ) ) ;
#5471=VECTOR ( 'NONE', #16136, 1000.000000000000227 ) ;
#5479=ADVANCED_FACE ( 'NONE', ( #1364 ), #7593, .T. ) ;
#5498=EDGE_LOOP ( 'NONE', ( #4980, #14689, #7232, #6679 ) ) ;
#5519=DIRECTION ( 'NONE',  ( 0.000000000000000000, 0.000000000000000000, 1.000000000000000000 ) ) ;
#5532=EDGE_CURVE ( 'NONE', #16978, #16737, #12264, .T. ) ;
#5557=CARTESIAN_POINT ( 'NONE',  ( -156.4179374840092862, -52.02840013024096066, 60.00000000000000000 ) ) ;
#5576=EDGE_LOOP ( 'NONE', ( #7626, #17569, #4274, #4395 ) ) ;
#5581=FACE_OUTER_BOUND ( 'NONE', #14740, .T. ) ;
#5590=FACE_OUTER_BOUND ( 'NONE', #5576, .T. ) ;
#5593=CARTESIAN_POINT ( 'NONE',  ( 128.2779226595531270, 102.2982297021113141, 60.00000000000000000 ) ) ;
#5625=DIRECTION ( 'NONE',  ( -0.000000000000000000, -0.000000000000000000, -1.000000000000000000 ) ) ;
#5639=AXIS2_PLACEMENT_3D ( 'NONE', #7350, #10218, #19445 ) ;
#5645=CARTESIAN_POINT ( 'NONE',  ( 0.000000000000000000, 0.000000000000000000, 60.00000000000000000 ) ) ;
#5661=DIRECTION ( 'NONE',  ( -0.000000000000000000, -0.000000000000000000, -1.000000000000000000 ) ) ;
#5675=EDGE_CURVE ( 'NONE', #4234, #2109, #20125, .T. ) ;
#5681=EDGE_LOOP ( 'NONE', ( #5425, #11818, #5065, #4733 ) ) ;
#5708=DIRECTION ( 'NONE',  ( 0.000000000000000000, 0.000000000000000000, 1.000000000000000000 ) ) ;
#5719=DIRECTION ( 'NONE',  ( -1.000000000000000000, 0.000000000000000000, 0.000000000000000000 ) ) ;
#5731=CYLINDRICAL_SURFACE ( 'NONE', #14969, 15.91767397667354800 ) ;
#5749=CIRCLE ( 'NONE', #16211, 15.91767397667354089 ) ;
#5776=ORIENTED_EDGE ( 'NONE', *, *, #1850, .F. ) ;
#5790=EDGE_LOOP ( 'NONE', ( #8970, #8483, #14543, #4606 ) ) ;
#5795=CARTESIAN_POINT ( 'NONE',  ( 78.68887634719573043, -147.8252249328912740, 60.00000000000000000 ) ) ;
#5796=FACE_OUTER_BOUND ( 'NONE', #16439, .T. ) ;
#5801=ORIENTED_EDGE ( 'NONE', *, *, #10832, .T. ) ;
#5818=CARTESIAN_POINT ( 'NONE',  ( 0.000000000000000000, 164.0736214083062805, 60.00000000000000000 ) ) ;
#5821=CARTESIAN_POINT ( 'NONE',  ( 0.000000000000000000, 164.0736214083062805, 49.99999999999999289 ) ) ;
#5823=CARTESIAN_POINT ( 'NONE',  ( 79.05640494598117129, -127.4758205975433327, 49.99999999999999289 ) ) ;
#5853=CARTESIAN_POINT ( 'NONE',  ( -79.05640494597940915, -127.4758205975444270, 60.00000000000000000 ) ) ;
#5856=VECTOR ( 'NONE', #14308, 1000.000000000000227 ) ;
#5908=ORIENTED_EDGE ( 'NONE', *, *, #2975, .F. ) ;
#5918=AXIS2_PLACEMENT_3D ( 'NONE', #7723, #13963, #3135 ) ;
#5968=CARTESIAN_POINT ( 'NONE',  ( 0.000000000000000000, 0.000000000000000000, 49.99999999999999289 ) ) ;
#5987=EDGE_CURVE ( 'NONE', #3620, #6087, #1674, .T. ) ;
#5988=AXIS2_PLACEMENT_3D ( 'NONE', #12458, #12360, #15545 ) ;
#6032=VECTOR ( 'NONE', #14986, 1000.000000000000000 ) ;
#6037=DIRECTION ( 'NONE',  ( -1.000000000000000000, 0.000000000000000000, 0.000000000000000000 ) ) ;
#6063=LINE ( 'NONE', #12068, #5008 ) ;
#6068=ORIENTED_EDGE ( 'NONE', *, *, #18801, .T. ) ;
#6073=DIRECTION ( 'NONE',  ( 0.000000000000000000, 0.000000000000000000, 1.000000000000000000 ) ) ;
#6083=CARTESIAN_POINT ( 'NONE',  ( -63.68887634719364144, -147.8252249328922687, 60.00000000000000000 ) ) ;
#6087=VERTEX_POINT ( 'NONE', #10967 ) ;
#6090=VECTOR ( 'NONE', #13617, 1000.000000000000227 ) ;
#6115=VERTEX_POINT ( 'NONE', #13170 ) ;
#6125=CARTESIAN_POINT ( 'NONE',  ( -150.0000000000000284, 0.000000000000000000, 60.00000000000000000 ) ) ;
#6127=AXIS2_PLACEMENT_3D ( 'NONE', #5821, #13577, #12042 ) ;
#6129=CARTESIAN_POINT ( 'NONE',  ( -87.10655032386719654, -147.8252249328922687, 60.00000000000000000 ) ) ;
#6144=VECTOR ( 'NONE', #19755, 1000.000000000000114 ) ;
#6153=CIRCLE ( 'NONE', #10060, 7.500000000000008882 ) ;
#6186=DIRECTION ( 'NONE',  ( -1.000000000000000000, 0.000000000000000000, 0.000000000000000000 ) ) ;
#6197=EDGE_CURVE ( 'NONE', #9011, #14411, #8776, .T. ) ;
#6230=VERTEX_POINT ( 'NONE', #6129 ) ;
#6251=CARTESIAN_POINT ( 'NONE',  ( -148.9554720520392834, -17.67108784863415138, 60.00000000000000000 ) ) ;
#6281=EDGE_CURVE ( 'NONE', #6717, #12028, #9019, .T. ) ;
#6285=EDGE_CURVE ( 'NONE', #17700, #8237, #1519, .T. ) ;
#6290=LINE ( 'NONE', #136, #8230 ) ;
#6301=ADVANCED_FACE ( 'NONE', ( #17484 ), #8054, .F. ) ;
#6320=CIRCLE ( 'NONE', #17749, 150.0000000000000284 ) ;
#6341=CARTESIAN_POINT ( 'NONE',  ( -15.91767397667354800, 164.0736214083062805, 49.99999999999999289 ) ) ;
#6367=CARTESIAN_POINT ( 'NONE',  ( -85.53020504959707182, -140.9188050298390067, 60.00000000000000000 ) ) ;
#6369=ADVANCED_FACE ( 'NONE', ( #11526 ), #12956, .F. ) ;
#6370=ORIENTED_EDGE ( 'NONE', *, *, #7341, .F. ) ;
#6423=EDGE_CURVE ( 'NONE', #13125, #9217, #3949, .T. ) ;
#6429=DIRECTION ( 'NONE',  ( 0.000000000000000000, 0.000000000000000000, 1.000000000000000000 ) ) ;
#6432=ORIENTED_EDGE ( 'NONE', *, *, #16130, .T. ) ;
#6434=DIRECTION ( 'NONE',  ( -0.000000000000000000, -0.000000000000000000, -1.000000000000000000 ) ) ;
#6442=CARTESIAN_POINT ( 'NONE',  ( 0.000000000000000000, 0.000000000000000000, 60.00000000000000000 ) ) ;
#6462=VERTEX_POINT ( 'NONE', #5795 ) ;
#6504=LINE ( 'NONE', #4659, #9941 ) ;
#6557=DIRECTION ( 'NONE',  ( 0.000000000000000000, 0.000000000000000000, 1.000000000000000000 ) ) ;
#6569=LINE ( 'NONE', #10946, #11966 ) ;
#6571=CIRCLE ( 'NONE', #7863, 150.0000000000000284 ) ;
#6572=CARTESIAN_POINT ( 'NONE',  ( 0.000000000000000000, 0.000000000000000000, 60.00000000000000000 ) ) ;
#6577=ORIENTED_EDGE ( 'NONE', *, *, #15894, .F. ) ;
#6615=DIRECTION ( 'NONE',  ( 0.000000000000000000, 0.000000000000000000, 1.000000000000000000 ) ) ;
#6631=ORIENTED_EDGE ( 'NONE', *, *, #5121, .F. ) ;
#6654=CARTESIAN_POINT ( 'NONE',  ( 120.7779226595530986, 102.2982297021113141, 60.00000000000000000 ) ) ;
#6672=EDGE_LOOP ( 'NONE', ( #4056, #14230, #918, #12943 ) ) ;
#6676=VERTEX_POINT ( 'NONE', #9364 ) ;
#6679=ORIENTED_EDGE ( 'NONE', *, *, #11610, .F. ) ;
#6700=VERTEX_POINT ( 'NONE', #57 ) ;
#6717=VERTEX_POINT ( 'NONE', #10478 ) ;
#6719=ORIENTED_EDGE ( 'NONE', *, *, #13494, .F. ) ;
#6728=PLANE ( 'NONE',  #5391 ) ;
#6742=VECTOR ( 'NONE', #4373, 1000.000000000000000 ) ;
#6750=CARTESIAN_POINT ( 'NONE',  ( 7.500000000000008882, 164.0736214083062805, 49.99999999999999289 ) ) ;
#6767=AXIS2_PLACEMENT_3D ( 'NONE', #12658, #5204, #18920 ) ;
#6770=CARTESIAN_POINT ( 'NONE',  ( 15.91767397667354089, 149.1530343478547422, 60.00000000000000000 ) ) ;
#6777=ORIENTED_EDGE ( 'NONE', *, *, #5251, .T. ) ;
#6806=EDGE_CURVE ( 'NONE', #11084, #10879, #1897, .T. ) ;
#6820=CIRCLE ( 'NONE', #15335, 15.91767397667355510 ) ;
#6942=LINE ( 'NONE', #3764, #9908 ) ;
#6943=ORIENTED_EDGE ( 'NONE', *, *, #17547, .F. ) ;
#6955=DIRECTION ( 'NONE',  ( -0.000000000000000000, -0.000000000000000000, -1.000000000000000000 ) ) ;
#6959=CYLINDRICAL_SURFACE ( 'NONE', #5639, 15.91767397667354089 ) ;
#6977=CARTESIAN_POINT ( 'NONE',  ( 0.000000000000000000, 0.000000000000000000, 60.00000000000000000 ) ) ;
#6979=EDGE_CURVE ( 'NONE', #3938, #16337, #3015, .T. ) ;
#6981=AXIS2_PLACEMENT_3D ( 'NONE', #11564, #5625, #2168 ) ;
#6982=EDGE_CURVE ( 'NONE', #14304, #8041, #6290, .T. ) ;
#6991=CIRCLE ( 'NONE', #16785, 7.500000000000007105 ) ;
#7010=PRODUCT_DEFINITION_CONTEXT ( 'detailed design', #2931, 'design' ) ;
#7060=CARTESIAN_POINT ( 'NONE',  ( -63.68887634719364144, -147.8252249328922687, 60.00000000000000000 ) ) ;
#7069=ORIENTED_EDGE ( 'NONE', *, *, #2486, .F. ) ;
#7083=CYLINDRICAL_SURFACE ( 'NONE', #3996, 15.91767397667354800 ) ;
#7091=SHAPE_REPRESENTATION_RELATIONSHIP ( 'NONE' , 'NONE' ,  #7558, #1643 ) ;
#7098=DIRECTION ( 'NONE',  ( 1.000000000000000000, 0.000000000000000000, 0.000000000000000000 ) ) ;
#7117=VERTEX_POINT ( 'NONE', #11675 ) ;
#7157=VECTOR ( 'NONE', #6434, 1000.000000000000000 ) ;
#7167=CARTESIAN_POINT ( 'NONE',  ( -71.18887634719365565, -147.8252249328922687, 60.00000000000000000 ) ) ;
#7170=VERTEX_POINT ( 'NONE', #17732 ) ;
#7181=EDGE_CURVE ( 'NONE', #13002, #1681, #19463, .T. ) ;
#7190=CARTESIAN_POINT ( 'NONE',  ( 135.7779226595531270, 102.2982297021113141, 60.00000000000000000 ) ) ;
#7191=ORIENTED_EDGE ( 'NONE', *, *, #17655, .T. ) ;
#7194=CIRCLE ( 'NONE', #15702, 15.91767397667354089 ) ;
#7217=DIRECTION ( 'NONE',  ( 0.6234898018587429203, -0.7818314824680223651, 0.000000000000000000 ) ) ;
#7225=DIRECTION ( 'NONE',  ( -0.000000000000000000, -0.000000000000000000, -1.000000000000000000 ) ) ;
#7232=ORIENTED_EDGE ( 'NONE', *, *, #10789, .T. ) ;
#7247=DIRECTION ( 'NONE',  ( 1.000000000000000000, 0.000000000000000000, 0.000000000000000000 ) ) ;
#7276=FACE_OUTER_BOUND ( 'NONE', #3453, .T. ) ;
#7281=DIRECTION ( 'NONE',  ( -0.000000000000000000, -0.000000000000000000, -1.000000000000000000 ) ) ;
#7288=ORIENTED_EDGE ( 'NONE', *, *, #18109, .T. ) ;
#7294=ORIENTED_EDGE ( 'NONE', *, *, #2975, .T. ) ;
#7302=ORIENTED_EDGE ( 'NONE', *, *, #19446, .F. ) ;
#7322=AXIS2_PLACEMENT_3D ( 'NONE', #18005, #16274, #3973 ) ;
#7341=EDGE_CURVE ( 'NONE', #13125, #1887, #12487, .T. ) ;
#7350=CARTESIAN_POINT ( 'NONE',  ( -71.18887634719365565, -147.8252249328922687, 60.00000000000000000 ) ) ;
#7420=CARTESIAN_POINT ( 'NONE',  ( 128.2779226595531270, 102.2982297021113141, 60.00000000000000000 ) ) ;
#7425=CARTESIAN_POINT ( 'NONE',  ( 15.91767397667354800, 164.0736214083062805, 60.00000000000000000 ) ) ;
#7434=CIRCLE ( 'NONE', #18563, 15.91767397667354089 ) ;
#7460=ORIENTED_EDGE ( 'NONE', *, *, #7736, .T. ) ;
#7468=SURFACE_STYLE_USAGE ( .BOTH. , #107 ) ;
#7489=EDGE_CURVE ( 'NONE', #3695, #16332, #4615, .T. ) ;
#7520=DIRECTION ( 'NONE',  ( -1.000000000000000000, 0.000000000000000000, 0.000000000000000000 ) ) ;
#7526=DIRECTION ( 'NONE',  ( 0.000000000000000000, 0.000000000000000000, 1.000000000000000000 ) ) ;
#7538=FACE_OUTER_BOUND ( 'NONE', #3341, .T. ) ;
#7540=CARTESIAN_POINT ( 'NONE',  ( 1.396592535537253342E-14, 0.000000000000000000, 60.00000000000000000 ) ) ;
#7542=CARTESIAN_POINT ( 'NONE',  ( 15.91767397667354089, 149.1530343478547422, 60.00000000000000000 ) ) ;
#7551=LINE ( 'NONE', #6341, #13251 ) ;
#7552=ORIENTED_EDGE ( 'NONE', *, *, #12778, .F. ) ;
#7558=SHAPE_REPRESENTATION ( 'Back Cover', ( #18639 ), #12 ) ;
#7560=ORIENTED_EDGE ( 'NONE', *, *, #15369, .F. ) ;
#7563=ORIENTED_EDGE ( 'NONE', *, *, #9079, .F. ) ;
#7565=DIRECTION ( 'NONE',  ( 1.000000000000000000, 0.000000000000000000, 0.000000000000000000 ) ) ;
#7566=VECTOR ( 'NONE', #5181, 1000.000000000000114 ) ;
#7569=CARTESIAN_POINT ( 'NONE',  ( 0.000000000000000000, 0.000000000000000000, 60.00000000000000000 ) ) ;
#7591=ADVANCED_FACE ( 'NONE', ( #615 ), #14629, .F. ) ;
#7593=CYLINDRICAL_SURFACE ( 'NONE', #833, 150.0000000000000284 ) ;
#7614=CARTESIAN_POINT ( 'NONE',  ( 71.18887634719571622, -147.8252249328912740, 49.99999999999999289 ) ) ;
#7626=ORIENTED_EDGE ( 'NONE', *, *, #4247, .F. ) ;
#7671=ADVANCED_FACE ( 'NONE', ( #277 ), #11214, .F. ) ;
#7682=ORIENTED_EDGE ( 'NONE', *, *, #18231, .F. ) ;
#7694=CIRCLE ( 'NONE', #1150, 150.0000000000000284 ) ;
#7705=EDGE_CURVE ( 'NONE', #7117, #4629, #12829, .T. ) ;
#7723=CARTESIAN_POINT ( 'NONE',  ( -159.9599531637108782, -36.50981547337168109, 60.00000000000000000 ) ) ;
#7728=LINE ( 'NONE', #13969, #18501 ) ;
#7729=EDGE_LOOP ( 'NONE', ( #1133, #706, #3491, #7560 ) ) ;
#7736=EDGE_CURVE ( 'NONE', #9812, #6115, #773, .T. ) ;
#7737=CARTESIAN_POINT ( 'NONE',  ( 167.4599531637113330, -36.50981547336952104, 49.99999999999999289 ) ) ;
#7785=EDGE_CURVE ( 'NONE', #1681, #1353, #3699, .T. ) ;
#7799=ORIENTED_EDGE ( 'NONE', *, *, #8477, .T. ) ;
#7837=PRODUCT_DEFINITION_SHAPE ( 'NONE', 'NONE',  #3275 ) ;
#7852=CARTESIAN_POINT ( 'NONE',  ( 126.5370453525553671, 80.55045718954892209, 49.99999999999999289 ) ) ;
#7858=DIRECTION ( 'NONE',  ( -0.000000000000000000, -0.000000000000000000, -1.000000000000000000 ) ) ;
#7863=AXIS2_PLACEMENT_3D ( 'NONE', #19243, #5519, #16370 ) ;
#7869=FACE_OUTER_BOUND ( 'NONE', #11820, .T. ) ;
#7890=EDGE_CURVE ( 'NONE', #20169, #19329, #12495, .T. ) ;
#7912=EDGE_CURVE ( 'NONE', #10504, #17700, #6320, .T. ) ;
#7920=CARTESIAN_POINT ( 'NONE',  ( 15.91767397667354089, 149.1530343478547422, 60.00000000000000000 ) ) ;
#7943=FACE_BOUND ( 'NONE', #3642, .T. ) ;
#7947=ORIENTED_EDGE ( 'NONE', *, *, #16413, .T. ) ;
#7968=ORIENTED_EDGE ( 'NONE', *, *, #3401, .F. ) ;
#7977=EDGE_CURVE ( 'NONE', #6462, #1353, #3101, .T. ) ;
#8007=EDGE_CURVE ( 'NONE', #4788, #10, #11170, .T. ) ;
#8009=CARTESIAN_POINT ( 'NONE',  ( -56.84754764479025368, -154.7316448359455308, 49.99999999999999289 ) ) ;
#8015=ORIENTED_EDGE ( 'NONE', *, *, #17243, .F. ) ;
#8023=CARTESIAN_POINT ( 'NONE',  ( 163.5019688434126977, -20.99123081650019884, 60.00000000000000000 ) ) ;
#8024=DIRECTION ( 'NONE',  ( 0.000000000000000000, 0.000000000000000000, 1.000000000000000000 ) ) ;
#8027=DIRECTION ( 'NONE',  ( 0.000000000000000000, 0.000000000000000000, 1.000000000000000000 ) ) ;
#8041=VERTEX_POINT ( 'NONE', #14450 ) ;
#8051=VECTOR ( 'NONE', #10403, 1000.000000000000000 ) ;
#8054=CYLINDRICAL_SURFACE ( 'NONE', #3490, 7.500000000000008882 ) ;
#8056=FACE_OUTER_BOUND ( 'NONE', #1806, .T. ) ;
#8057=LINE ( 'NONE', #19120, #11262 ) ;
#8076=DIRECTION ( 'NONE',  ( 1.000000000000000000, 0.000000000000000000, 0.000000000000000000 ) ) ;
#8087=VECTOR ( 'NONE', #3732, 1000.000000000000114 ) ;
#8104=CARTESIAN_POINT ( 'NONE',  ( -159.9599531637108782, -36.50981547337168109, 60.00000000000000000 ) ) ;
#8118=ORIENTED_EDGE ( 'NONE', *, *, #15585, .F. ) ;
#8134=CARTESIAN_POINT ( 'NONE',  ( 126.5370453525553671, 80.55045718954892209, 60.00000000000000000 ) ) ;
#8180=LINE ( 'NONE', #5316, #173 ) ;
#8199=AXIS2_PLACEMENT_3D ( 'NONE', #19318, #5400, #11529 ) ;
#8210=DIRECTION ( 'NONE',  ( 0.9749279121818261729, -0.2225209339563031519, 0.000000000000000000 ) ) ;
#8213=LINE ( 'NONE', #17835, #9318 ) ;
#8230=VECTOR ( 'NONE', #8210, 1000.000000000000114 ) ;
#8237=VERTEX_POINT ( 'NONE', #12881 ) ;
#8243=VECTOR ( 'NONE', #18738, 1000.000000000000000 ) ;
#8280=CARTESIAN_POINT ( 'NONE',  ( 156.4179374840099683, -52.02840013023883614, 60.00000000000000000 ) ) ;
#8281=CARTESIAN_POINT ( 'NONE',  ( 1.396592535537253342E-14, 0.000000000000000000, 49.99999999999999289 ) ) ;
#8308=EDGE_CURVE ( 'NONE', #16337, #3938, #1828, .T. ) ;
#8317=AXIS2_PLACEMENT_3D ( 'NONE', #14571, #3723, #7098 ) ;
#8334=EDGE_LOOP ( 'NONE', ( #2680, #8692, #10949, #18153 ) ) ;
#8353=ORIENTED_EDGE ( 'NONE', *, *, #1850, .T. ) ;
#8356=CARTESIAN_POINT ( 'NONE',  ( 159.9599531637113330, -36.50981547336952104, 60.00000000000000000 ) ) ;
#8357=VECTOR ( 'NONE', #20009, 1000.000000000000000 ) ;
#8385=DIRECTION ( 'NONE',  ( -1.000000000000000000, 0.000000000000000000, 0.000000000000000000 ) ) ;
#8399=ORIENTED_EDGE ( 'NONE', *, *, #3897, .T. ) ;
#8407=CARTESIAN_POINT ( 'NONE',  ( -163.5019688434124419, -20.99123081650240863, 49.99999999999999289 ) ) ;
#8412=VECTOR ( 'NONE', #10101, 1000.000000000000000 ) ;
#8415=EDGE_CURVE ( 'NONE', #2269, #12253, #1195, .T. ) ;
#8416=CARTESIAN_POINT ( 'NONE',  ( 0.000000000000000000, 0.000000000000000000, 0.000000000000000000 ) ) ;
#8427=ORIENTED_EDGE ( 'NONE', *, *, #7785, .F. ) ;
#8444=ORIENTED_EDGE ( 'NONE', *, *, #18599, .T. ) ;
#8464=CARTESIAN_POINT ( 'NONE',  ( 126.5370453525553671, 80.55045718954892209, 60.00000000000000000 ) ) ;
#8477=EDGE_CURVE ( 'NONE', #9812, #17524, #9074, .T. ) ;
#8479=DIRECTION ( 'NONE',  ( -0.000000000000000000, -0.000000000000000000, -1.000000000000000000 ) ) ;
#8483=ORIENTED_EDGE ( 'NONE', *, *, #8415, .F. ) ;
#8486=DIRECTION ( 'NONE',  ( 0.000000000000000000, 0.000000000000000000, 1.000000000000000000 ) ) ;
#8502=ADVANCED_FACE ( 'NONE', ( #20228 ), #12447, .F. ) ;
#8510=ADVANCED_FACE ( 'NONE', ( #3558 ), #6728, .F. ) ;
#8571=AXIS2_PLACEMENT_3D ( 'NONE', #6572, #14337, #19053 ) ;
#8574=DIRECTION ( 'NONE',  ( 4.650550193362991910E-16, 1.000000000000000000, 0.000000000000000000 ) ) ;
#8590=CARTESIAN_POINT ( 'NONE',  ( 50.37374754117451658, -141.2886604036503115, 60.00000000000000000 ) ) ;
#8615=EDGE_CURVE ( 'NONE', #16737, #16978, #17200, .T. ) ;
#8618=AXIS2_PLACEMENT_3D ( 'NONE', #9549, #18974, #232 ) ;
#8644=ORIENTED_EDGE ( 'NONE', *, *, #14588, .F. ) ;
#8692=ORIENTED_EDGE ( 'NONE', *, *, #1907, .F. ) ;
#8709=DIRECTION ( 'NONE',  ( -1.000000000000000000, 0.000000000000000000, 0.000000000000000000 ) ) ;
#8711=ORIENTED_EDGE ( 'NONE', *, *, #1584, .F. ) ;
#8712=CARTESIAN_POINT ( 'NONE',  ( 128.2779226595531270, 102.2982297021113141, 60.00000000000000000 ) ) ;
#8735=EDGE_CURVE ( 'NONE', #17877, #11084, #10977, .T. ) ;
#8738=EDGE_LOOP ( 'NONE', ( #12076, #13457 ) ) ;
#8742=CARTESIAN_POINT ( 'NONE',  ( -71.18887634719365565, -147.8252249328922687, 60.00000000000000000 ) ) ;
#8748=EDGE_CURVE ( 'NONE', #17524, #9946, #8801, .T. ) ;
#8776=LINE ( 'NONE', #11929, #8051 ) ;
#8798=CARTESIAN_POINT ( 'NONE',  ( -167.4599531637108782, -36.50981547337168109, 60.00000000000000000 ) ) ;
#8799=VERTEX_POINT ( 'NONE', #19744 ) ;
#8801=LINE ( 'NONE', #13596, #17152 ) ;
#8882=DIRECTION ( 'NONE',  ( 1.000000000000000000, 0.000000000000000000, 0.000000000000000000 ) ) ;
#8912=AXIS2_PLACEMENT_3D ( 'NONE', #11634, #17597, #3674 ) ;
#8925=DIRECTION ( 'NONE',  ( -0.9749279121818261729, 0.2225209339563031519, 0.000000000000000000 ) ) ;
#8940=LINE ( 'NONE', #18263, #6032 ) ;
#8949=DIRECTION ( 'NONE',  ( 0.000000000000000000, 0.000000000000000000, 1.000000000000000000 ) ) ;
#8950=CARTESIAN_POINT ( 'NONE',  ( 106.6880305650188347, 105.4403344747995988, 60.00000000000000000 ) ) ;
#8955=LINE ( 'NONE', #4463, #8357 ) ;
#8956=ORIENTED_EDGE ( 'NONE', *, *, #18540, .F. ) ;
#8960=EDGE_LOOP ( 'NONE', ( #16798, #1381, #3797, #19489 ) ) ;
#8970=ORIENTED_EDGE ( 'NONE', *, *, #1509, .T. ) ;
#9008=CARTESIAN_POINT ( 'NONE',  ( 118.3534152657848608, 114.7431683447366595, 49.99999999999999289 ) ) ;
#9011=VERTEX_POINT ( 'NONE', #9710 ) ;
#9018=CARTESIAN_POINT ( 'NONE',  ( 7.500000000000008882, 164.0736214083062805, 60.00000000000000000 ) ) ;
#9019=CIRCLE ( 'NONE', #1529, 7.500000000000008882 ) ;
#9033=CARTESIAN_POINT ( 'NONE',  ( 1.396592535537253342E-14, 0.000000000000000000, 60.00000000000000000 ) ) ;
#9051=DIRECTION ( 'NONE',  ( -1.000000000000000000, 0.000000000000000000, 0.000000000000000000 ) ) ;
#9059=ORIENTED_EDGE ( 'NONE', *, *, #7912, .T. ) ;
#9060=EDGE_LOOP ( 'NONE', ( #6432, #11368, #4069, #18346 ) ) ;
#9061=DIRECTION ( 'NONE',  ( 1.000000000000000000, 0.000000000000000000, 0.000000000000000000 ) ) ;
#9063=ORIENTED_EDGE ( 'NONE', *, *, #15369, .T. ) ;
#9074=LINE ( 'NONE', #7542, #6742 ) ;
#9075=CARTESIAN_POINT ( 'NONE',  ( -159.9599531637108782, -36.50981547337168109, 60.00000000000000000 ) ) ;
#9076=VERTEX_POINT ( 'NONE', #14524 ) ;
#9079=EDGE_CURVE ( 'NONE', #12028, #2362, #8180, .T. ) ;
#9093=EDGE_CURVE ( 'NONE', #17191, #11184, #5416, .T. ) ;
#9107=DIRECTION ( 'NONE',  ( 0.000000000000000000, 0.000000000000000000, 1.000000000000000000 ) ) ;
#9123=CARTESIAN_POINT ( 'NONE',  ( 50.37374754117451658, -141.2886604036503115, 60.00000000000000000 ) ) ;
#9173=CARTESIAN_POINT ( 'NONE',  ( 79.05640494598117129, -127.4758205975433327, 60.00000000000000000 ) ) ;
#9183=VECTOR ( 'NONE', #5163, 1000.000000000000000 ) ;
#9187=CIRCLE ( 'NONE', #1349, 150.0000000000000284 ) ;
#9211=FACE_OUTER_BOUND ( 'NONE', #5498, .T. ) ;
#9217=VERTEX_POINT ( 'NONE', #4374 ) ;
#9223=ADVANCED_FACE ( 'NONE', ( #3967 ), #19715, .F. ) ;
#9242=EDGE_CURVE ( 'NONE', #10879, #10504, #18296, .T. ) ;
#9256=ORIENTED_EDGE ( 'NONE', *, *, #9242, .T. ) ;
#9286=ORIENTED_EDGE ( 'NONE', *, *, #11719, .F. ) ;
#9315=CARTESIAN_POINT ( 'NONE',  ( 50.37374754117451658, -141.2886604036503115, 60.00000000000000000 ) ) ;
#9318=VECTOR ( 'NONE', #3515, 1000.000000000000227 ) ;
#9324=DIRECTION ( 'NONE',  ( -0.4338837391175509040, -0.9009688679024224767, 0.000000000000000000 ) ) ;
#9359=LINE ( 'NONE', #8023, #12542 ) ;
#9364=CARTESIAN_POINT ( 'NONE',  ( -78.68887634719368407, -147.8252249328922687, 49.99999999999999289 ) ) ;
#9365=CARTESIAN_POINT ( 'NONE',  ( 163.5019688434126977, -20.99123081650019884, 60.00000000000000000 ) ) ;
#9373=CARTESIAN_POINT ( 'NONE',  ( 120.7779226595530986, 102.2982297021113141, 49.99999999999999289 ) ) ;
#9380=EDGE_CURVE ( 'NONE', #698, #3700, #9391, .T. ) ;
#9391=LINE ( 'NONE', #6125, #7157 ) ;
#9415=EDGE_CURVE ( 'NONE', #698, #599, #3569, .T. ) ;
#9420=FILL_AREA_STYLE_COLOUR ( '', #3738 ) ;
#9459=ORIENTED_EDGE ( 'NONE', *, *, #1903, .F. ) ;
#9474=EDGE_LOOP ( 'NONE', ( #13523, #6777, #18282, #2965 ) ) ;
#9487=DIRECTION ( 'NONE',  ( -0.9009688679024207003, 0.4338837391175549563, 0.000000000000000000 ) ) ;
#9492=ORIENTED_EDGE ( 'NONE', *, *, #17547, .T. ) ;
#9531=EDGE_CURVE ( 'NONE', #17394, #8237, #1926, .T. ) ;
#9536=ORIENTED_EDGE ( 'NONE', *, *, #12400, .T. ) ;
#9544=CARTESIAN_POINT ( 'NONE',  ( 141.8714406926368099, -48.70825716237082759, 49.99999999999999289 ) ) ;
#9549=CARTESIAN_POINT ( 'NONE',  ( 1.396592535537253342E-14, 0.000000000000000000, 49.99999999999999289 ) ) ;
#9566=DIRECTION ( 'NONE',  ( 1.000000000000000000, 0.000000000000000000, 0.000000000000000000 ) ) ;
#9572=AXIS2_PLACEMENT_3D ( 'NONE', #8590, #14828, #17911 ) ;
#9580=VECTOR ( 'NONE', #15783, 1000.000000000000000 ) ;
#9591=DIRECTION ( 'NONE',  ( 1.000000000000000000, 0.000000000000000000, 0.000000000000000000 ) ) ;
#9621=ORIENTED_EDGE ( 'NONE', *, *, #10622, .F. ) ;
#9645=FACE_OUTER_BOUND ( 'NONE', #4811, .T. ) ;
#9676=VECTOR ( 'NONE', #11551, 1000.000000000000000 ) ;
#9693=DIRECTION ( 'NONE',  ( -0.000000000000000000, -0.000000000000000000, -1.000000000000000000 ) ) ;
#9709=EDGE_LOOP ( 'NONE', ( #2075, #16929, #4597, #16947 ) ) ;
#9710=CARTESIAN_POINT ( 'NONE',  ( -163.5019688434124419, -20.99123081650240863, 60.00000000000000000 ) ) ;
#9717=CARTESIAN_POINT ( 'NONE',  ( -17.49999999999999289, 0.000000000000000000, 60.00000000000000000 ) ) ;
#9794=DIRECTION ( 'NONE',  ( -0.000000000000000000, -0.000000000000000000, -1.000000000000000000 ) ) ;
#9809=CIRCLE ( 'NONE', #13069, 7.500000000000007105 ) ;
#9812=VERTEX_POINT ( 'NONE', #7920 ) ;
#9901=DIRECTION ( 'NONE',  ( 0.000000000000000000, 0.000000000000000000, 1.000000000000000000 ) ) ;
#9908=VECTOR ( 'NONE', #19229, 1000.000000000000000 ) ;
#9934=ORIENTED_EDGE ( 'NONE', *, *, #8615, .T. ) ;
#9938=ORIENTED_EDGE ( 'NONE', *, *, #8615, .F. ) ;
#9941=VECTOR ( 'NONE', #3327, 1000.000000000000114 ) ;
#9946=VERTEX_POINT ( 'NONE', #254 ) ;
#9948=FACE_OUTER_BOUND ( 'NONE', #2663, .T. ) ;
#9956=CARTESIAN_POINT ( 'NONE',  ( 56.84754764479241373, -154.7316448359447634, 49.99999999999999289 ) ) ;
#9968=CARTESIAN_POINT ( 'NONE',  ( -87.10655032386719654, -147.8252249328922687, 49.99999999999999289 ) ) ;
#10012=DIRECTION ( 'NONE',  ( -0.7818314824680226982, -0.6234898018587423651, 0.000000000000000000 ) ) ;
#10013=CLOSED_SHELL ( 'NONE', ( #4955, #4776, #19780, #12525, #7591, #6301, #12271, #18548, #15011, #16597, #11996, #847, #5479, #6369, #14614, #13087, #2015, #2874, #16021, #7671, #1782, #15932, #3243, #8502, #3229, #18775, #20053, #2769, #10896, #11731, #2302, #12765, #17270, #17920, #13220, #8510, #4749, #16146, #9223, #2177, #18251, #2172, #10965 ) ) ;
#10014=LINE ( 'NONE', #13165, #3407 ) ;
#10060=AXIS2_PLACEMENT_3D ( 'NONE', #15081, #13541, #1063 ) ;
#10073=CYLINDRICAL_SURFACE ( 'NONE', #12109, 7.500000000000020428 ) ;
#10078=CIRCLE ( 'NONE', #1247, 15.91767397667354089 ) ;
#10087=CARTESIAN_POINT ( 'NONE',  ( 15.91767397667354089, 149.1530343478547422, 60.00000000000000000 ) ) ;
#10091=ORIENTED_EDGE ( 'NONE', *, *, #15498, .F. ) ;
#10101=DIRECTION ( 'NONE',  ( -0.000000000000000000, -0.000000000000000000, -1.000000000000000000 ) ) ;
#10143=PRODUCT_DEFINITION_FORMATION_WITH_SPECIFIED_SOURCE ( 'ANY', '', #4, .NOT_KNOWN. ) ;
#10172=CARTESIAN_POINT ( 'NONE',  ( 163.5019688434126977, -20.99123081650019884, 60.00000000000000000 ) ) ;
#10182=CARTESIAN_POINT ( 'NONE',  ( -56.84754764479025368, -154.7316448359455308, 49.99999999999999289 ) ) ;
#10187=ORIENTED_EDGE ( 'NONE', *, *, #6982, .F. ) ;
#10189=DIRECTION ( 'NONE',  ( -0.000000000000000000, -0.000000000000000000, -1.000000000000000000 ) ) ;
#10196=VECTOR ( 'NONE', #5209, 1000.000000000000000 ) ;
#10206=CARTESIAN_POINT ( 'NONE',  ( 128.2779226595531270, 102.2982297021113141, 49.99999999999999289 ) ) ;
#10218=DIRECTION ( 'NONE',  ( -0.000000000000000000, -0.000000000000000000, -1.000000000000000000 ) ) ;
#10243=VERTEX_POINT ( 'NONE', #10765 ) ;
#10252=DIRECTION ( 'NONE',  ( 0.000000000000000000, 0.000000000000000000, 1.000000000000000000 ) ) ;
#10279=CYLINDRICAL_SURFACE ( 'NONE', #2553, 7.500000000000020428 ) ;
#10281=AXIS2_PLACEMENT_3D ( 'NONE', #9075, #2445, #11735 ) ;
#10287=DIRECTION ( 'NONE',  ( -0.000000000000000000, -0.000000000000000000, -1.000000000000000000 ) ) ;
#10338=DIRECTION ( 'NONE',  ( 1.000000000000000000, 0.000000000000000000, 0.000000000000000000 ) ) ;
#10347=DIRECTION ( 'NONE',  ( -0.000000000000000000, -0.000000000000000000, -1.000000000000000000 ) ) ;
#10355=EDGE_CURVE ( 'NONE', #11184, #16332, #4523, .T. ) ;
#10363=AXIS2_PLACEMENT_3D ( 'NONE', #8712, #6615, #10338 ) ;
#10382=EDGE_CURVE ( 'NONE', #17163, #14304, #19528, .T. ) ;
#10403=DIRECTION ( 'NONE',  ( -0.000000000000000000, -0.000000000000000000, -1.000000000000000000 ) ) ;
#10465=EDGE_CURVE ( 'NONE', #17524, #3620, #13998, .T. ) ;
#10478=CARTESIAN_POINT ( 'NONE',  ( 7.500000000000008882, 164.0736214083062805, 60.00000000000000000 ) ) ;
#10482=UNCERTAINTY_MEASURE_WITH_UNIT (LENGTH_MEASURE( 1.000000000000000082E-05 ), #20157, 'distance_accuracy_value', 'NONE');
#10484=CARTESIAN_POINT ( 'NONE',  ( 0.000000000000000000, 0.000000000000000000, 60.00000000000000000 ) ) ;
#10503=CARTESIAN_POINT ( 'NONE',  ( -79.05640494597940915, -127.4758205975444270, 49.99999999999999289 ) ) ;
#10504=VERTEX_POINT ( 'NONE', #10604 ) ;
#10507=DIRECTION ( 'NONE',  ( 1.000000000000000000, 0.000000000000000000, 0.000000000000000000 ) ) ;
#10510=ORIENTED_EDGE ( 'NONE', *, *, #984, .F. ) ;
#10515=DIRECTION ( 'NONE',  ( -0.000000000000000000, -0.000000000000000000, -1.000000000000000000 ) ) ;
#10546=AXIS2_PLACEMENT_3D ( 'NONE', #4926, #6557, #403 ) ;
#10556=CARTESIAN_POINT ( 'NONE',  ( 163.5019688434126977, -20.99123081650019884, 49.99999999999999289 ) ) ;
#10574=DIRECTION ( 'NONE',  ( 1.000000000000000000, 0.000000000000000000, 0.000000000000000000 ) ) ;
#10589=CARTESIAN_POINT ( 'NONE',  ( 0.000000000000000000, 0.000000000000000000, 49.99999999999999289 ) ) ;
#10598=VERTEX_POINT ( 'NONE', #12555 ) ;
#10604=CARTESIAN_POINT ( 'NONE',  ( 148.9554720520395392, -17.67108784863215476, 49.99999999999999289 ) ) ;
#10618=ORIENTED_EDGE ( 'NONE', *, *, #7181, .F. ) ;
#10622=EDGE_CURVE ( 'NONE', #17815, #9217, #14095, .T. ) ;
#10630=( NAMED_UNIT ( * ) PLANE_ANGLE_UNIT ( ) SI_UNIT ( $, .RADIAN. ) );
#10655=DIRECTION ( 'NONE',  ( -1.000000000000000000, 0.000000000000000000, 0.000000000000000000 ) ) ;
#10665=LINE ( 'NONE', #6083, #9183 ) ;
#10695=CARTESIAN_POINT ( 'NONE',  ( 152.4599531637113330, -36.50981547336952104, 49.99999999999999289 ) ) ;
#10697=ORIENTED_EDGE ( 'NONE', *, *, #17308, .T. ) ;
#10735=AXIS2_PLACEMENT_3D ( 'NONE', #16836, #8949, #17982 ) ;
#10748=CARTESIAN_POINT ( 'NONE',  ( 156.4179374840099683, -52.02840013023883614, 60.00000000000000000 ) ) ;
#10760=DIRECTION ( 'NONE',  ( 0.000000000000000000, 0.000000000000000000, 1.000000000000000000 ) ) ;
#10765=CARTESIAN_POINT ( 'NONE',  ( -167.4599531637108782, -36.50981547337168109, 49.99999999999999289 ) ) ;
#10768=FACE_OUTER_BOUND ( 'NONE', #889, .T. ) ;
#10789=EDGE_CURVE ( 'NONE', #3700, #3934, #17305, .T. ) ;
#10795=CARTESIAN_POINT ( 'NONE',  ( 71.18887634719571622, -147.8252249328912740, 49.99999999999999289 ) ) ;
#10832=EDGE_CURVE ( 'NONE', #599, #9011, #19413, .T. ) ;
#10848=ORIENTED_EDGE ( 'NONE', *, *, #18801, .F. ) ;
#10862=EDGE_CURVE ( 'NONE', #17330, #5317, #3458, .T. ) ;
#10879=VERTEX_POINT ( 'NONE', #13444 ) ;
#10896=ADVANCED_FACE ( 'NONE', ( #5796 ), #13348, .T. ) ;
#10909=LINE ( 'NONE', #20223, #16228 ) ;
#10915=DIRECTION ( 'NONE',  ( 0.4338837391175643932, -0.9009688679024161484, 0.000000000000000000 ) ) ;
#10923=AXIS2_PLACEMENT_3D ( 'NONE', #16513, #2799, #10655 ) ;
#10927=ORIENTED_EDGE ( 'NONE', *, *, #17779, .T. ) ;
#10928=FACE_OUTER_BOUND ( 'NONE', #19347, .T. ) ;
#10946=CARTESIAN_POINT ( 'NONE',  ( -15.91767397667355510, 149.1530343478547422, 60.00000000000000000 ) ) ;
#10949=ORIENTED_EDGE ( 'NONE', *, *, #17298, .F. ) ;
#10953=EDGE_CURVE ( 'NONE', #13849, #5317, #2909, .T. ) ;
#10965=ADVANCED_FACE ( 'NONE', ( #5590 ), #1174, .F. ) ;
#10967=CARTESIAN_POINT ( 'NONE',  ( -15.91767397667354800, 164.0736214083062805, 49.99999999999999289 ) ) ;
#10969=EDGE_CURVE ( 'NONE', #4491, #9076, #20000, .T. ) ;
#10977=CIRCLE ( 'NONE', #11932, 15.91767397667354089 ) ;
#10994=CARTESIAN_POINT ( 'NONE',  ( -159.9599531637108782, -36.50981547337168109, 49.99999999999999289 ) ) ;
#11007=VERTEX_POINT ( 'NONE', #3231 ) ;
#11010=FACE_BOUND ( 'NONE', #17803, .T. ) ;
#11016=CARTESIAN_POINT ( 'NONE',  ( 0.000000000000000000, 0.000000000000000000, 60.00000000000000000 ) ) ;
#11060=AXIS2_PLACEMENT_3D ( 'NONE', #15629, #6429, #1617 ) ;
#11075=DIRECTION ( 'NONE',  ( -0.000000000000000000, -0.000000000000000000, -1.000000000000000000 ) ) ;
#11082=ORIENTED_EDGE ( 'NONE', *, *, #15894, .T. ) ;
#11084=VERTEX_POINT ( 'NONE', #9365 ) ;
#11129=CARTESIAN_POINT ( 'NONE',  ( 0.000000000000000000, 164.0736214083062805, 60.00000000000000000 ) ) ;
#11153=CARTESIAN_POINT ( 'NONE',  ( -159.9599531637108782, -36.50981547337168109, 60.00000000000000000 ) ) ;
#11170=LINE ( 'NONE', #328, #19075 ) ;
#11184=VERTEX_POINT ( 'NONE', #11305 ) ;
#11196=CARTESIAN_POINT ( 'NONE',  ( 163.5019688434126977, -20.99123081650019884, 60.00000000000000000 ) ) ;
#11214=PLANE ( 'NONE',  #1400 ) ;
#11220=ORIENTED_EDGE ( 'NONE', *, *, #7890, .T. ) ;
#11233=DIRECTION ( 'NONE',  ( -0.000000000000000000, -0.000000000000000000, -1.000000000000000000 ) ) ;
#11243=MECHANICAL_DESIGN_GEOMETRIC_PRESENTATION_REPRESENTATION('',(#19433),#1113);
#11262=VECTOR ( 'NONE', #3264, 1000.000000000000000 ) ;
#11284=DIRECTION ( 'NONE',  ( 0.000000000000000000, 0.000000000000000000, 1.000000000000000000 ) ) ;
#11300=VECTOR ( 'NONE', #12136, 1000.000000000000000 ) ;
#11305=CARTESIAN_POINT ( 'NONE',  ( 17.50000000000001776, 2.143131898507868643E-15, 49.99999999999999289 ) ) ;
#11312=AXIS2_PLACEMENT_3D ( 'NONE', #7614, #2822, #10574 ) ;
#11346=EDGE_LOOP ( 'NONE', ( #18371, #2082 ) ) ;
#11349=FACE_BOUND ( 'NONE', #14684, .T. ) ;
#11368=ORIENTED_EDGE ( 'NONE', *, *, #16744, .F. ) ;
#11415=ORIENTED_EDGE ( 'NONE', *, *, #10953, .F. ) ;
#11418=EDGE_CURVE ( 'NONE', #15200, #14483, #19641, .T. ) ;
#11428=DIRECTION ( 'NONE',  ( -1.000000000000000000, 0.000000000000000000, 0.000000000000000000 ) ) ;
#11437=LINE ( 'NONE', #3756, #8412 ) ;
#11446=VECTOR ( 'NONE', #4431, 1000.000000000000114 ) ;
#11447=DIRECTION ( 'NONE',  ( -0.000000000000000000, -0.000000000000000000, -1.000000000000000000 ) ) ;
#11455=DIRECTION ( 'NONE',  ( -0.000000000000000000, -0.000000000000000000, -1.000000000000000000 ) ) ;
#11465=ORIENTED_EDGE ( 'NONE', *, *, #20028, .F. ) ;
#11472=ORIENTED_EDGE ( 'NONE', *, *, #8007, .F. ) ;
#11512=ORIENTED_EDGE ( 'NONE', *, *, #7489, .T. ) ;
#11518=DIRECTION ( 'NONE',  ( 0.000000000000000000, 0.000000000000000000, 1.000000000000000000 ) ) ;
#11521=ORIENTED_EDGE ( 'NONE', *, *, #10862, .F. ) ;
#11526=FACE_OUTER_BOUND ( 'NONE', #17294, .T. ) ;
#11529=DIRECTION ( 'NONE',  ( -1.000000000000000000, 0.000000000000000000, 0.000000000000000000 ) ) ;
#11547=CIRCLE ( 'NONE', #12842, 7.500000000000007105 ) ;
#11551=DIRECTION ( 'NONE',  ( -0.000000000000000000, -0.000000000000000000, -1.000000000000000000 ) ) ;
#11564=CARTESIAN_POINT ( 'NONE',  ( 1.396592535537253342E-14, 0.000000000000000000, 60.00000000000000000 ) ) ;
#11586=ORIENTED_EDGE ( 'NONE', *, *, #16412, .T. ) ;
#11610=EDGE_CURVE ( 'NONE', #599, #3934, #18516, .T. ) ;
#11634=CARTESIAN_POINT ( 'NONE',  ( -159.9599531637108782, -36.50981547337168109, 49.99999999999999289 ) ) ;
#11656=ORIENTED_EDGE ( 'NONE', *, *, #11418, .F. ) ;
#11657=DIRECTION ( 'NONE',  ( 1.000000000000000000, 0.000000000000000000, 0.000000000000000000 ) ) ;
#11659=VERTEX_POINT ( 'NONE', #6750 ) ;
#11674=AXIS2_PLACEMENT_3D ( 'NONE', #5593, #9901, #19605 ) ;
#11675=CARTESIAN_POINT ( 'NONE',  ( -50.37374754117255549, -141.2886604036510221, 49.99999999999999289 ) ) ;
#11683=ORIENTED_EDGE ( 'NONE', *, *, #9380, .F. ) ;
#11685=ORIENTED_EDGE ( 'NONE', *, *, #8735, .T. ) ;
#11701=ORIENTED_EDGE ( 'NONE', *, *, #258, .F. ) ;
#11712=ORIENTED_EDGE ( 'NONE', *, *, #5675, .T. ) ;
#11719=EDGE_CURVE ( 'NONE', #11007, #16337, #402, .T. ) ;
#11731=ADVANCED_FACE ( 'NONE', ( #600 ), #3577, .F. ) ;
#11734=DIRECTION ( 'NONE',  ( 1.000000000000000000, 0.000000000000000000, 0.000000000000000000 ) ) ;
#11735=DIRECTION ( 'NONE',  ( -1.000000000000000000, 0.000000000000000000, 0.000000000000000000 ) ) ;
#11740=DIRECTION ( 'NONE',  ( 0.000000000000000000, 0.000000000000000000, 1.000000000000000000 ) ) ;
#11741=LINE ( 'NONE', #3880, #344 ) ;
#11750=DIRECTION ( 'NONE',  ( 0.000000000000000000, 0.000000000000000000, 1.000000000000000000 ) ) ;
#11767=DIRECTION ( 'NONE',  ( -0.000000000000000000, -0.000000000000000000, -1.000000000000000000 ) ) ;
#11796=ORIENTED_EDGE ( 'NONE', *, *, #12108, .F. ) ;
#11798=ORIENTED_EDGE ( 'NONE', *, *, #15585, .T. ) ;
#11818=ORIENTED_EDGE ( 'NONE', *, *, #18038, .F. ) ;
#11820=EDGE_LOOP ( 'NONE', ( #17571, #13767, #95, #10510, #7302, #813, #12418, #17596, #13557, #10848, #7552, #10187, #11701, #18900, #3869, #8118, #19582, #2240, #4014, #7682, #11656, #5776, #9621, #20070, #17451, #5203, #18589 ) ) ;
#11835=FACE_OUTER_BOUND ( 'NONE', #9709, .T. ) ;
#11847=ORIENTED_EDGE ( 'NONE', *, *, #4247, .T. ) ;
#11907=EDGE_CURVE ( 'NONE', #19329, #4788, #6820, .T. ) ;
#11913=FACE_OUTER_BOUND ( 'NONE', #8334, .T. ) ;
#11929=CARTESIAN_POINT ( 'NONE',  ( -163.5019688434124419, -20.99123081650240863, 60.00000000000000000 ) ) ;
#11932=AXIS2_PLACEMENT_3D ( 'NONE', #16783, #15341, #7565 ) ;
#11946=CIRCLE ( 'NONE', #17210, 150.0000000000000284 ) ;
#11966=VECTOR ( 'NONE', #4827, 1000.000000000000000 ) ;
#11980=AXIS2_PLACEMENT_3D ( 'NONE', #6442, #12664, #389 ) ;
#11981=AXIS2_PLACEMENT_3D ( 'NONE', #18769, #4646, #4328 ) ;
#11996=ADVANCED_FACE ( 'NONE', ( #1305, #7943, #17272, #7538, #11010, #4470, #20224, #176 ), #18703, .T. ) ;
#12015=CARTESIAN_POINT ( 'NONE',  ( 0.000000000000000000, 0.000000000000000000, 60.00000000000000000 ) ) ;
#12017=EDGE_CURVE ( 'NONE', #6230, #18743, #18909, .T. ) ;
#12028=VERTEX_POINT ( 'NONE', #18490 ) ;
#12037=CIRCLE ( 'NONE', #4183, 17.50000000000000355 ) ;
#12040=AXIS2_PLACEMENT_3D ( 'NONE', #1257, #13939, #8925 ) ;
#12042=DIRECTION ( 'NONE',  ( 1.000000000000000000, 0.000000000000000000, 0.000000000000000000 ) ) ;
#12068=CARTESIAN_POINT ( 'NONE',  ( -156.4179374840092862, -52.02840013024096066, 60.00000000000000000 ) ) ;
#12076=ORIENTED_EDGE ( 'NONE', *, *, #14588, .T. ) ;
#12080=FACE_OUTER_BOUND ( 'NONE', #5281, .T. ) ;
#12108=EDGE_CURVE ( 'NONE', #6717, #11659, #18546, .T. ) ;
#12109=AXIS2_PLACEMENT_3D ( 'NONE', #16324, #2405, #856 ) ;
#12136=DIRECTION ( 'NONE',  ( -0.000000000000000000, -0.000000000000000000, -1.000000000000000000 ) ) ;
#12155=ORIENTED_EDGE ( 'NONE', *, *, #19219, .T. ) ;
#12178=AXIS2_PLACEMENT_3D ( 'NONE', #17712, #6955, #8385 ) ;
#12253=VERTEX_POINT ( 'NONE', #4371 ) ;
#12264=CIRCLE ( 'NONE', #17194, 7.500000000000020428 ) ;
#12271=ADVANCED_FACE ( 'NONE', ( #15314 ), #1307, .F. ) ;
#12356=AXIS2_PLACEMENT_3D ( 'NONE', #5818, #4071, #7247 ) ;
#12358=CIRCLE ( 'NONE', #18232, 15.91767397667354089 ) ;
#12360=DIRECTION ( 'NONE',  ( -0.000000000000000000, -0.000000000000000000, -1.000000000000000000 ) ) ;
#12371=AXIS2_PLACEMENT_3D ( 'NONE', #12015, #1289, #9051 ) ;
#12380=CARTESIAN_POINT ( 'NONE',  ( 118.3534152657848608, 114.7431683447366595, 60.00000000000000000 ) ) ;
#12400=EDGE_CURVE ( 'NONE', #11659, #2362, #18547, .T. ) ;
#12418=ORIENTED_EDGE ( 'NONE', *, *, #4734, .F. ) ;
#12439=AXIS2_PLACEMENT_3D ( 'NONE', #15090, #16544, #19602 ) ;
#12447=PLANE ( 'NONE',  #4739 ) ;
#12458=CARTESIAN_POINT ( 'NONE',  ( 159.9599531637113330, -36.50981547336952104, 60.00000000000000000 ) ) ;
#12487=CIRCLE ( 'NONE', #14462, 150.0000000000000284 ) ;
#12488=EDGE_CURVE ( 'NONE', #20112, #7117, #16536, .T. ) ;
#12495=LINE ( 'NONE', #9123, #5025 ) ;
#12504=AXIS2_PLACEMENT_3D ( 'NONE', #377, #14494, #12851 ) ;
#12520=ORIENTED_EDGE ( 'NONE', *, *, #8748, .F. ) ;
#12522=DIRECTION ( 'NONE',  ( 0.7818314824680222541, 0.6234898018587428092, 0.000000000000000000 ) ) ;
#12525=ADVANCED_FACE ( 'NONE', ( #5581 ), #10279, .F. ) ;
#12542=VECTOR ( 'NONE', #3124, 1000.000000000000000 ) ;
#12550=ORIENTED_EDGE ( 'NONE', *, *, #3897, .F. ) ;
#12555=CARTESIAN_POINT ( 'NONE',  ( -152.4599531637108498, -36.50981547337168109, 49.99999999999999289 ) ) ;
#12563=ORIENTED_EDGE ( 'NONE', *, *, #6806, .F. ) ;
#12571=ORIENTED_EDGE ( 'NONE', *, *, #7489, .F. ) ;
#12608=CYLINDRICAL_SURFACE ( 'NONE', #4610, 15.91767397667354089 ) ;
#12627=DIRECTION ( 'NONE',  ( 0.000000000000000000, 0.000000000000000000, 1.000000000000000000 ) ) ;
#12646=ORIENTED_EDGE ( 'NONE', *, *, #18038, .T. ) ;
#12657=CIRCLE ( 'NONE', #11674, 15.91767397667354089 ) ;
#12658=CARTESIAN_POINT ( 'NONE',  ( -148.9554720520392834, -17.67108784863415138, 60.00000000000000000 ) ) ;
#12664=DIRECTION ( 'NONE',  ( -0.000000000000000000, -0.000000000000000000, -1.000000000000000000 ) ) ;
#12666=EDGE_CURVE ( 'NONE', #2362, #11659, #6153, .T. ) ;
#12667=ORIENTED_EDGE ( 'NONE', *, *, #2673, .F. ) ;
#12677=VERTEX_POINT ( 'NONE', #17041 ) ;
#12699=VECTOR ( 'NONE', #12884, 1000.000000000000000 ) ;
#12702=ORIENTED_EDGE ( 'NONE', *, *, #14786, .T. ) ;
#12703=DIRECTION ( 'NONE',  ( -0.4338837391175643932, 0.9009688679024161484, 0.000000000000000000 ) ) ;
#12740=CARTESIAN_POINT ( 'NONE',  ( 0.000000000000000000, 0.000000000000000000, 60.00000000000000000 ) ) ;
#12765=ADVANCED_FACE ( 'NONE', ( #20095 ), #3025, .F. ) ;
#12778=EDGE_CURVE ( 'NONE', #8041, #12677, #7434, .T. ) ;
#12792=CARTESIAN_POINT ( 'NONE',  ( -78.68887634719368407, -147.8252249328922687, 60.00000000000000000 ) ) ;
#12823=ORIENTED_EDGE ( 'NONE', *, *, #12778, .T. ) ;
#12829=CIRCLE ( 'NONE', #12504, 150.0000000000000284 ) ;
#12831=DIRECTION ( 'NONE',  ( 1.000000000000000000, 0.000000000000000000, 0.000000000000000000 ) ) ;
#12842=AXIS2_PLACEMENT_3D ( 'NONE', #2861, #18618, #18412 ) ;
#12851=DIRECTION ( 'NONE',  ( 1.000000000000000000, 0.000000000000000000, 0.000000000000000000 ) ) ;
#12856=ORIENTED_EDGE ( 'NONE', *, *, #9093, .T. ) ;
#12859=ORIENTED_EDGE ( 'NONE', *, *, #3500, .T. ) ;
#12861=CARTESIAN_POINT ( 'NONE',  ( 0.000000000000000000, 0.000000000000000000, 49.99999999999999289 ) ) ;
#12873=VERTEX_POINT ( 'NONE', #1690 ) ;
#12881=CARTESIAN_POINT ( 'NONE',  ( 138.2024300533213932, 89.85329105948596862, 49.99999999999999289 ) ) ;
#12884=DIRECTION ( 'NONE',  ( -0.000000000000000000, -0.000000000000000000, -1.000000000000000000 ) ) ;
#12943=ORIENTED_EDGE ( 'NONE', *, *, #8748, .T. ) ;
#12956=PLANE ( 'NONE',  #6767 ) ;
#12982=CARTESIAN_POINT ( 'NONE',  ( 56.84754764479241373, -154.7316448359447634, 60.00000000000000000 ) ) ;
#13002=VERTEX_POINT ( 'NONE', #16415 ) ;
#13030=VECTOR ( 'NONE', #5000, 1000.000000000000000 ) ;
#13043=EDGE_LOOP ( 'NONE', ( #11465, #15769 ) ) ;
#13058=CYLINDRICAL_SURFACE ( 'NONE', #8199, 7.500000000000020428 ) ;
#13064=EDGE_LOOP ( 'NONE', ( #3195, #941 ) ) ;
#13069=AXIS2_PLACEMENT_3D ( 'NONE', #17511, #5030, #8076 ) ;
#13087=ADVANCED_FACE ( 'NONE', ( #16014 ), #1998, .F. ) ;
#13125=VERTEX_POINT ( 'NONE', #16808 ) ;
#13129=EDGE_CURVE ( 'NONE', #2720, #6700, #16707, .T. ) ;
#13142=ORIENTED_EDGE ( 'NONE', *, *, #19604, .F. ) ;
#13149=DIRECTION ( 'NONE',  ( 0.000000000000000000, 0.000000000000000000, 1.000000000000000000 ) ) ;
#13159=CIRCLE ( 'NONE', #8912, 7.500000000000007105 ) ;
#13164=DIRECTION ( 'NONE',  ( -0.6234898018587424762, 0.7818314824680228092, 0.000000000000000000 ) ) ;
#13165=CARTESIAN_POINT ( 'NONE',  ( 15.91767397667354089, 149.1530343478547422, 49.99999999999999289 ) ) ;
#13170=CARTESIAN_POINT ( 'NONE',  ( 15.91767397667354089, 149.1530343478547422, 49.99999999999999289 ) ) ;
#13196=DIRECTION ( 'NONE',  ( -1.000000000000000000, 0.000000000000000000, 0.000000000000000000 ) ) ;
#13220=ADVANCED_FACE ( 'NONE', ( #1018 ), #5731, .T. ) ;
#13227=EDGE_LOOP ( 'NONE', ( #6068, #17350, #12563, #900 ) ) ;
#13251=VECTOR ( 'NONE', #19930, 1000.000000000000000 ) ;
#13261=DIRECTION ( 'NONE',  ( 0.000000000000000000, 0.000000000000000000, 1.000000000000000000 ) ) ;
#13287=CARTESIAN_POINT ( 'NONE',  ( -148.9554720520392834, -17.67108784863415138, 60.00000000000000000 ) ) ;
#13293=CYLINDRICAL_SURFACE ( 'NONE', #4964, 150.0000000000000284 ) ;
#13297=VECTOR ( 'NONE', #2702, 1000.000000000000000 ) ;
#13317=ORIENTED_EDGE ( 'NONE', *, *, #16292, .T. ) ;
#13335=AXIS2_PLACEMENT_3D ( 'NONE', #7420, #7225, #7520 ) ;
#13348=CYLINDRICAL_SURFACE ( 'NONE', #12371, 150.0000000000000284 ) ;
#13376=ORIENTED_EDGE ( 'NONE', *, *, #16410, .F. ) ;
#13414=LINE ( 'NONE', #19665, #13821 ) ;
#13416=CARTESIAN_POINT ( 'NONE',  ( -56.84754764479025368, -154.7316448359455308, 60.00000000000000000 ) ) ;
#13423=DIRECTION ( 'NONE',  ( 1.000000000000000000, 0.000000000000000000, 0.000000000000000000 ) ) ;
#13444=CARTESIAN_POINT ( 'NONE',  ( 148.9554720520395392, -17.67108784863215476, 60.00000000000000000 ) ) ;
#13457=ORIENTED_EDGE ( 'NONE', *, *, #10355, .T. ) ;
#13470=EDGE_CURVE ( 'NONE', #10598, #10243, #13159, .T. ) ;
#13482=ORIENTED_EDGE ( 'NONE', *, *, #1472, .F. ) ;
#13494=EDGE_CURVE ( 'NONE', #6700, #7117, #6942, .T. ) ;
#13500=DIRECTION ( 'NONE',  ( 1.000000000000000000, 0.000000000000000000, 0.000000000000000000 ) ) ;
#13504=LINE ( 'NONE', #741, #6144 ) ;
#13523=ORIENTED_EDGE ( 'NONE', *, *, #19604, .T. ) ;
#13537=CIRCLE ( 'NONE', #4744, 17.50000000000000355 ) ;
#13541=DIRECTION ( 'NONE',  ( 0.000000000000000000, 0.000000000000000000, 1.000000000000000000 ) ) ;
#13554=DIRECTION ( 'NONE',  ( -0.4338837391175643932, 0.9009688679024161484, 0.000000000000000000 ) ) ;
#13557=ORIENTED_EDGE ( 'NONE', *, *, #7912, .F. ) ;
#13577=DIRECTION ( 'NONE',  ( 0.000000000000000000, 0.000000000000000000, 1.000000000000000000 ) ) ;
#13596=CARTESIAN_POINT ( 'NONE',  ( 15.91767397667354800, 164.0736214083062805, 60.00000000000000000 ) ) ;
#13603=DIRECTION ( 'NONE',  ( 0.000000000000000000, 0.000000000000000000, 1.000000000000000000 ) ) ;
#13613=( NAMED_UNIT ( * ) SI_UNIT ( $, .STERADIAN. ) SOLID_ANGLE_UNIT ( ) );
#13617=DIRECTION ( 'NONE',  ( 0.9749279121818226201, 0.2225209339563185562, 0.000000000000000000 ) ) ;
#13669=AXIS2_PLACEMENT_3D ( 'NONE', #16115, #16018, #4877 ) ;
#13694=DIRECTION ( 'NONE',  ( -1.000000000000000000, 0.000000000000000000, 0.000000000000000000 ) ) ;
#13720=VECTOR ( 'NONE', #7858, 1000.000000000000000 ) ;
#13726=DIRECTION ( 'NONE',  ( 1.000000000000000000, 0.000000000000000000, 0.000000000000000000 ) ) ;
#13742=ORIENTED_EDGE ( 'NONE', *, *, #12666, .F. ) ;
#13760=DIRECTION ( 'NONE',  ( 1.000000000000000000, 0.000000000000000000, 0.000000000000000000 ) ) ;
#13767=ORIENTED_EDGE ( 'NONE', *, *, #16130, .F. ) ;
#13768=DIRECTION ( 'NONE',  ( 0.000000000000000000, 0.000000000000000000, 1.000000000000000000 ) ) ;
#13780=CARTESIAN_POINT ( 'NONE',  ( 106.6880305650188347, 105.4403344747995988, 60.00000000000000000 ) ) ;
#13812=CARTESIAN_POINT ( 'NONE',  ( -15.91767397667355510, 149.1530343478547422, 60.00000000000000000 ) ) ;
#13821=VECTOR ( 'NONE', #5661, 1000.000000000000000 ) ;
#13835=CARTESIAN_POINT ( 'NONE',  ( 0.000000000000000000, 0.000000000000000000, 60.00000000000000000 ) ) ;
#13849=VERTEX_POINT ( 'NONE', #7737 ) ;
#13886=EDGE_LOOP ( 'NONE', ( #14878, #18827, #13742, #7563 ) ) ;
#13912=DIRECTION ( 'NONE',  ( -0.000000000000000000, -0.000000000000000000, -1.000000000000000000 ) ) ;
#13914=CARTESIAN_POINT ( 'NONE',  ( 0.000000000000000000, 0.000000000000000000, 60.00000000000000000 ) ) ;
#13927=ORIENTED_EDGE ( 'NONE', *, *, #5532, .F. ) ;
#13934=VECTOR ( 'NONE', #10189, 1000.000000000000000 ) ;
#13939=DIRECTION ( 'NONE',  ( 0.2225209339563031519, 0.9749279121818261729, -0.000000000000000000 ) ) ;
#13943=PLANE ( 'NONE',  #11981 ) ;
#13963=DIRECTION ( 'NONE',  ( 0.000000000000000000, 0.000000000000000000, 1.000000000000000000 ) ) ;
#13969=CARTESIAN_POINT ( 'NONE',  ( 85.53020504959901871, -140.9188050298377846, 49.99999999999999289 ) ) ;
#13981=VECTOR ( 'NONE', #718, 1000.000000000000227 ) ;
#13984=EDGE_LOOP ( 'NONE', ( #3983, #9536 ) ) ;
#13998=CIRCLE ( 'NONE', #12356, 15.91767397667354800 ) ;
#14001=AXIS2_PLACEMENT_3D ( 'NONE', #17355, #12627, #12831 ) ;
#14004=ORIENTED_EDGE ( 'NONE', *, *, #17746, .F. ) ;
#14017=LINE ( 'NONE', #9315, #473 ) ;
#14049=DIRECTION ( 'NONE',  ( 1.000000000000000000, 0.000000000000000000, 0.000000000000000000 ) ) ;
#14082=CIRCLE ( 'NONE', #16697, 7.500000000000020428 ) ;
#14087=CARTESIAN_POINT ( 'NONE',  ( -87.10655032386719654, -147.8252249328922687, 60.00000000000000000 ) ) ;
#14092=DIRECTION ( 'NONE',  ( 0.000000000000000000, 0.000000000000000000, 1.000000000000000000 ) ) ;
#14095=LINE ( 'NONE', #1822, #5856 ) ;
#14140=CARTESIAN_POINT ( 'NONE',  ( 0.000000000000000000, 0.000000000000000000, 49.99999999999999289 ) ) ;
#14151=AXIS2_PLACEMENT_3D ( 'NONE', #17770, #11518, #5196 ) ;
#14204=DIRECTION ( 'NONE',  ( 1.000000000000000000, 0.000000000000000000, 0.000000000000000000 ) ) ;
#14208=ORIENTED_EDGE ( 'NONE', *, *, #262, .T. ) ;
#14230=ORIENTED_EDGE ( 'NONE', *, *, #5987, .F. ) ;
#14248=EDGE_CURVE ( 'NONE', #10, #16031, #13414, .T. ) ;
#14300=EDGE_LOOP ( 'NONE', ( #19682, #1610, #17651, #3702 ) ) ;
#14304=VERTEX_POINT ( 'NONE', #9544 ) ;
#14308=DIRECTION ( 'NONE',  ( 0.9749279121818226201, 0.2225209339563185562, 0.000000000000000000 ) ) ;
#14310=FACE_OUTER_BOUND ( 'NONE', #3160, .T. ) ;
#14337=DIRECTION ( 'NONE',  ( 0.000000000000000000, 0.000000000000000000, 1.000000000000000000 ) ) ;
#14346=VECTOR ( 'NONE', #10287, 1000.000000000000000 ) ;
#14360=DIRECTION ( 'NONE',  ( 1.000000000000000000, 0.000000000000000000, 0.000000000000000000 ) ) ;
#14391=ORIENTED_EDGE ( 'NONE', *, *, #7181, .T. ) ;
#14411=VERTEX_POINT ( 'NONE', #8407 ) ;
#14450=CARTESIAN_POINT ( 'NONE',  ( 156.4179374840099683, -52.02840013023883614, 49.99999999999999289 ) ) ;
#14462=AXIS2_PLACEMENT_3D ( 'NONE', #13914, #13603, #4098 ) ;
#14483=VERTEX_POINT ( 'NONE', #3606 ) ;
#14485=AXIS2_PLACEMENT_3D ( 'NONE', #92, #11233, #5015 ) ;
#14494=DIRECTION ( 'NONE',  ( 0.000000000000000000, 0.000000000000000000, 1.000000000000000000 ) ) ;
#14524=CARTESIAN_POINT ( 'NONE',  ( -175.8776271403844191, -36.50981547337168109, 49.99999999999999289 ) ) ;
#14543=ORIENTED_EDGE ( 'NONE', *, *, #15519, .F. ) ;
#14571=CARTESIAN_POINT ( 'NONE',  ( -71.18887634719365565, -147.8252249328922687, 49.99999999999999289 ) ) ;
#14588=EDGE_CURVE ( 'NONE', #16332, #11184, #17126, .T. ) ;
#14605=LINE ( 'NONE', #2606, #15180 ) ;
#14611=DIRECTION ( 'NONE',  ( 1.000000000000000000, 0.000000000000000000, 0.000000000000000000 ) ) ;
#14614=ADVANCED_FACE ( 'NONE', ( #9645 ), #1873, .T. ) ;
#14629=CYLINDRICAL_SURFACE ( 'NONE', #12178, 7.500000000000007105 ) ;
#14633=AXIS2_PLACEMENT_3D ( 'NONE', #7540, #20020, #16750 ) ;
#14684=EDGE_LOOP ( 'NONE', ( #2941, #205 ) ) ;
#14689=ORIENTED_EDGE ( 'NONE', *, *, #9380, .T. ) ;
#14732=LINE ( 'NONE', #18105, #13981 ) ;
#14740=EDGE_LOOP ( 'NONE', ( #9934, #7294, #18399, #12550 ) ) ;
#14745=AXIS2_PLACEMENT_3D ( 'NONE', #16714, #19484, #13423 ) ;
#14786=EDGE_CURVE ( 'NONE', #20169, #4629, #14017, .T. ) ;
#14805=ORIENTED_EDGE ( 'NONE', *, *, #7705, .T. ) ;
#14828=DIRECTION ( 'NONE',  ( 0.9009688679024152602, 0.4338837391175662805, -0.000000000000000000 ) ) ;
#14854=MANIFOLD_SOLID_BREP ( 'Boss-Extrude11', #10013 ) ;
#14870=FACE_OUTER_BOUND ( 'NONE', #17625, .T. ) ;
#14872=DIRECTION ( 'NONE',  ( 0.9749279121818255067, -0.2225209339563057331, 0.000000000000000000 ) ) ;
#14875=ORIENTED_EDGE ( 'NONE', *, *, #4870, .T. ) ;
#14878=ORIENTED_EDGE ( 'NONE', *, *, #20028, .T. ) ;
#14922=CARTESIAN_POINT ( 'NONE',  ( -15.91767397667354800, 164.0736214083062805, 60.00000000000000000 ) ) ;
#14931=DIRECTION ( 'NONE',  ( -0.4338837391175509040, -0.9009688679024224767, 0.000000000000000000 ) ) ;
#14954=AXIS2_PLACEMENT_3D ( 'NONE', #1107, #20039, #6037 ) ;
#14957=EDGE_LOOP ( 'NONE', ( #3601, #5288, #18520, #13317 ) ) ;
#14963=CARTESIAN_POINT ( 'NONE',  ( -156.4179374840092862, -52.02840013024096066, 60.00000000000000000 ) ) ;
#14969=AXIS2_PLACEMENT_3D ( 'NONE', #1326, #10515, #13694 ) ;
#14985=AXIS2_PLACEMENT_3D ( 'NONE', #3330, #8027, #19090 ) ;
#14986=DIRECTION ( 'NONE',  ( -0.000000000000000000, -0.000000000000000000, -1.000000000000000000 ) ) ;
#15010=EDGE_CURVE ( 'NONE', #9076, #17815, #5382, .T. ) ;
#15011=ADVANCED_FACE ( 'NONE', ( #11835 ), #17906, .T. ) ;
#15045=CIRCLE ( 'NONE', #5918, 7.500000000000007105 ) ;
#15050=CYLINDRICAL_SURFACE ( 'NONE', #18604, 150.0000000000000284 ) ;
#15081=CARTESIAN_POINT ( 'NONE',  ( 0.000000000000000000, 164.0736214083062805, 49.99999999999999289 ) ) ;
#15090=CARTESIAN_POINT ( 'NONE',  ( 128.2779226595531270, 102.2982297021113141, 60.00000000000000000 ) ) ;
#15112=ORIENTED_EDGE ( 'NONE', *, *, #1472, .T. ) ;
#15124=FACE_OUTER_BOUND ( 'NONE', #5681, .T. ) ;
#15127=CYLINDRICAL_SURFACE ( 'NONE', #14954, 7.500000000000020428 ) ;
#15129=EDGE_LOOP ( 'NONE', ( #3672, #20015 ) ) ;
#15133=ORIENTED_EDGE ( 'NONE', *, *, #10382, .T. ) ;
#15142=CARTESIAN_POINT ( 'NONE',  ( 85.53020504959901871, -140.9188050298377846, 49.99999999999999289 ) ) ;
#15180=VECTOR ( 'NONE', #18150, 1000.000000000000114 ) ;
#15200=VERTEX_POINT ( 'NONE', #10503 ) ;
#15282=EDGE_LOOP ( 'NONE', ( #17079, #17053, #10697, #25 ) ) ;
#15314=FACE_OUTER_BOUND ( 'NONE', #4619, .T. ) ;
#15326=CARTESIAN_POINT ( 'NONE',  ( -150.0000000000000284, 0.000000000000000000, 49.99999999999999289 ) ) ;
#15335=AXIS2_PLACEMENT_3D ( 'NONE', #1088, #5708, #4064 ) ;
#15341=DIRECTION ( 'NONE',  ( 0.000000000000000000, 0.000000000000000000, 1.000000000000000000 ) ) ;
#15345=FILL_AREA_STYLE ('',( #9420 ) ) ;
#15369=EDGE_CURVE ( 'NONE', #2720, #20112, #8057, .T. ) ;
#15387=ORIENTED_EDGE ( 'NONE', *, *, #11907, .T. ) ;
#15418=ORIENTED_EDGE ( 'NONE', *, *, #8007, .T. ) ;
#15437=CARTESIAN_POINT ( 'NONE',  ( 85.53020504959901871, -140.9188050298377846, 60.00000000000000000 ) ) ;
#15455=DIRECTION ( 'NONE',  ( -1.000000000000000000, 0.000000000000000000, 0.000000000000000000 ) ) ;
#15459=CARTESIAN_POINT ( 'NONE',  ( -159.9599531637108782, -36.50981547337168109, 49.99999999999999289 ) ) ;
#15461=AXIS2_PLACEMENT_3D ( 'NONE', #19324, #5406, #14611 ) ;
#15498=EDGE_CURVE ( 'NONE', #3695, #17191, #13537, .T. ) ;
#15519=EDGE_CURVE ( 'NONE', #16556, #2269, #14605, .T. ) ;
#15535=ORIENTED_EDGE ( 'NONE', *, *, #8308, .F. ) ;
#15537=DIRECTION ( 'NONE',  ( 0.000000000000000000, 0.000000000000000000, 1.000000000000000000 ) ) ;
#15542=AXIS2_PLACEMENT_3D ( 'NONE', #10206, #19619, #11734 ) ;
#15545=DIRECTION ( 'NONE',  ( -1.000000000000000000, 0.000000000000000000, 0.000000000000000000 ) ) ;
#15578=CARTESIAN_POINT ( 'NONE',  ( 78.68887634719573043, -147.8252249328912740, 60.00000000000000000 ) ) ;
#15585=EDGE_CURVE ( 'NONE', #4629, #4234, #8213, .T. ) ;
#15616=DIRECTION ( 'NONE',  ( 0.000000000000000000, 0.000000000000000000, 1.000000000000000000 ) ) ;
#15629=CARTESIAN_POINT ( 'NONE',  ( 0.000000000000000000, 0.000000000000000000, 60.00000000000000000 ) ) ;
#15644=LINE ( 'NONE', #1632, #13720 ) ;
#15649=CIRCLE ( 'NONE', #14985, 7.500000000000020428 ) ;
#15666=SURFACE_STYLE_FILL_AREA ( #15345 ) ;
#15681=ORIENTED_EDGE ( 'NONE', *, *, #14248, .T. ) ;
#15688=DIRECTION ( 'NONE',  ( 0.4338837391175662250, -0.9009688679024151492, 0.000000000000000000 ) ) ;
#15702=AXIS2_PLACEMENT_3D ( 'NONE', #11153, #3391, #15873 ) ;
#15716=ORIENTED_EDGE ( 'NONE', *, *, #987, .T. ) ;
#15733=DIRECTION ( 'NONE',  ( 1.000000000000000000, 0.000000000000000000, 0.000000000000000000 ) ) ;
#15736=DIRECTION ( 'NONE',  ( -0.000000000000000000, -0.000000000000000000, -1.000000000000000000 ) ) ;
#15753=FACE_BOUND ( 'NONE', #13064, .T. ) ;
#15769=ORIENTED_EDGE ( 'NONE', *, *, #6281, .F. ) ;
#15783=DIRECTION ( 'NONE',  ( -0.000000000000000000, -0.000000000000000000, -1.000000000000000000 ) ) ;
#15828=EDGE_LOOP ( 'NONE', ( #8015, #19285 ) ) ;
#15873=DIRECTION ( 'NONE',  ( 1.000000000000000000, 0.000000000000000000, 0.000000000000000000 ) ) ;
#15894=EDGE_CURVE ( 'NONE', #6700, #20169, #1390, .T. ) ;
#15930=ORIENTED_EDGE ( 'NONE', *, *, #6197, .T. ) ;
#15932=ADVANCED_FACE ( 'NONE', ( #18199 ), #1105, .F. ) ;
#16003=ORIENTED_EDGE ( 'NONE', *, *, #10969, .F. ) ;
#16014=FACE_OUTER_BOUND ( 'NONE', #14300, .T. ) ;
#16018=DIRECTION ( 'NONE',  ( -0.000000000000000000, -0.000000000000000000, -1.000000000000000000 ) ) ;
#16021=ADVANCED_FACE ( 'NONE', ( #15124 ), #6959, .T. ) ;
#16031=VERTEX_POINT ( 'NONE', #5823 ) ;
#16047=FACE_OUTER_BOUND ( 'NONE', #17602, .T. ) ;
#16115=CARTESIAN_POINT ( 'NONE',  ( -71.18887634719365565, -147.8252249328922687, 60.00000000000000000 ) ) ;
#16130=EDGE_CURVE ( 'NONE', #6087, #5083, #7551, .T. ) ;
#16136=DIRECTION ( 'NONE',  ( 0.4338837391175549563, 0.9009688679024205893, 0.000000000000000000 ) ) ;
#16145=DIRECTION ( 'NONE',  ( 1.000000000000000000, 0.000000000000000000, 0.000000000000000000 ) ) ;
#16146=ADVANCED_FACE ( 'NONE', ( #3267 ), #2037, .F. ) ;
#16211=AXIS2_PLACEMENT_3D ( 'NONE', #2206, #16518, #18144 ) ;
#16226=EDGE_LOOP ( 'NONE', ( #19306, #4888 ) ) ;
#16228=VECTOR ( 'NONE', #372, 1000.000000000000000 ) ;
#16261=APPLICATION_CONTEXT ( 'automotive_design' ) ;
#16272=CARTESIAN_POINT ( 'NONE',  ( 141.8714406926368099, -48.70825716237082759, 60.00000000000000000 ) ) ;
#16274=DIRECTION ( 'NONE',  ( 0.000000000000000000, 0.000000000000000000, 1.000000000000000000 ) ) ;
#16292=EDGE_CURVE ( 'NONE', #7170, #17700, #3859, .T. ) ;
#16300=DIRECTION ( 'NONE',  ( -0.000000000000000000, -0.000000000000000000, -1.000000000000000000 ) ) ;
#16324=CARTESIAN_POINT ( 'NONE',  ( 71.18887634719571622, -147.8252249328912740, 60.00000000000000000 ) ) ;
#16332=VERTEX_POINT ( 'NONE', #20005 ) ;
#16337=VERTEX_POINT ( 'NONE', #9373 ) ;
#16370=DIRECTION ( 'NONE',  ( 1.000000000000000000, 0.000000000000000000, 0.000000000000000000 ) ) ;
#16385=VECTOR ( 'NONE', #18550, 1000.000000000000000 ) ;
#16398=FACE_OUTER_BOUND ( 'NONE', #4940, .T. ) ;
#16410=EDGE_CURVE ( 'NONE', #2269, #9812, #17867, .T. ) ;
#16412=EDGE_CURVE ( 'NONE', #2109, #16031, #7728, .T. ) ;
#16413=EDGE_CURVE ( 'NONE', #6462, #13002, #18177, .T. ) ;
#16415=CARTESIAN_POINT ( 'NONE',  ( 63.68887634719569490, -147.8252249328912740, 60.00000000000000000 ) ) ;
#16438=DIRECTION ( 'NONE',  ( -0.000000000000000000, -0.000000000000000000, -1.000000000000000000 ) ) ;
#16439=EDGE_LOOP ( 'NONE', ( #9059, #2335, #6631, #9256 ) ) ;
#16446=CARTESIAN_POINT ( 'NONE',  ( -141.8714406926361562, -48.70825716237266079, 60.00000000000000000 ) ) ;
#16470=AXIS2_PLACEMENT_3D ( 'NONE', #8104, #442, #19170 ) ;
#16498=DIRECTION ( 'NONE',  ( -1.000000000000000000, 0.000000000000000000, 0.000000000000000000 ) ) ;
#16513=CARTESIAN_POINT ( 'NONE',  ( 0.000000000000000000, 0.000000000000000000, 60.00000000000000000 ) ) ;
#16518=DIRECTION ( 'NONE',  ( 0.000000000000000000, 0.000000000000000000, 1.000000000000000000 ) ) ;
#16521=DIRECTION ( 'NONE',  ( -0.2225209339563057609, -0.9749279121818256177, 0.000000000000000000 ) ) ;
#16536=LINE ( 'NONE', #10182, #5471 ) ;
#16544=DIRECTION ( 'NONE',  ( -0.000000000000000000, -0.000000000000000000, -1.000000000000000000 ) ) ;
#16556=VERTEX_POINT ( 'NONE', #12380 ) ;
#16597=ADVANCED_FACE ( 'NONE', ( #9211 ), #4203, .T. ) ;
#16612=VERTEX_POINT ( 'NONE', #13812 ) ;
#16626=EDGE_LOOP ( 'NONE', ( #19940, #14004 ) ) ;
#16645=VECTOR ( 'NONE', #14931, 1000.000000000000114 ) ;
#16669=CARTESIAN_POINT ( 'NONE',  ( -17.49999999999999289, 0.000000000000000000, 60.00000000000000000 ) ) ;
#16673=DIRECTION ( 'NONE',  ( 0.000000000000000000, 0.000000000000000000, 1.000000000000000000 ) ) ;
#16697=AXIS2_PLACEMENT_3D ( 'NONE', #10795, #17050, #13760 ) ;
#16699=( NAMED_UNIT ( * ) PLANE_ANGLE_UNIT ( ) SI_UNIT ( $, .RADIAN. ) );
#16700=AXIS2_PLACEMENT_3D ( 'NONE', #4855, #1778, #14360 ) ;
#16707=LINE ( 'NONE', #13416, #18927 ) ;
#16711=PLANE ( 'NONE',  #12040 ) ;
#16714=CARTESIAN_POINT ( 'NONE',  ( -71.18887634719365565, -147.8252249328922687, 49.99999999999999289 ) ) ;
#16735=CARTESIAN_POINT ( 'NONE',  ( -7.500000000000008882, 164.0736214083062805, 49.99999999999999289 ) ) ;
#16737=VERTEX_POINT ( 'NONE', #12792 ) ;
#16744=EDGE_CURVE ( 'NONE', #16612, #5083, #6569, .T. ) ;
#16750=DIRECTION ( 'NONE',  ( -1.000000000000000000, 0.000000000000000000, 0.000000000000000000 ) ) ;
#16783=CARTESIAN_POINT ( 'NONE',  ( 159.9599531637113330, -36.50981547336952104, 60.00000000000000000 ) ) ;
#16785=AXIS2_PLACEMENT_3D ( 'NONE', #798, #13261, #19523 ) ;
#16798=ORIENTED_EDGE ( 'NONE', *, *, #11418, .T. ) ;
#16808=CARTESIAN_POINT ( 'NONE',  ( -141.8714406926361562, -48.70825716237266079, 60.00000000000000000 ) ) ;
#16829=ORIENTED_EDGE ( 'NONE', *, *, #20100, .F. ) ;
#16836=CARTESIAN_POINT ( 'NONE',  ( 159.9599531637113330, -36.50981547336952104, 49.99999999999999289 ) ) ;
#16869=CARTESIAN_POINT ( 'NONE',  ( -71.18887634719365565, -147.8252249328922687, 49.99999999999999289 ) ) ;
#16892=CARTESIAN_POINT ( 'NONE',  ( 1.396592535537253342E-14, 0.000000000000000000, 60.00000000000000000 ) ) ;
#16929=ORIENTED_EDGE ( 'NONE', *, *, #10969, .T. ) ;
#16947=ORIENTED_EDGE ( 'NONE', *, *, #4419, .F. ) ;
#16978=VERTEX_POINT ( 'NONE', #7060 ) ;
#16987=VERTEX_POINT ( 'NONE', #2550 ) ;
#17032=EDGE_CURVE ( 'NONE', #18743, #20112, #1888, .T. ) ;
#17041=CARTESIAN_POINT ( 'NONE',  ( 163.5019688434126977, -20.99123081650019884, 49.99999999999999289 ) ) ;
#17042=ORIENTED_EDGE ( 'NONE', *, *, #13129, .T. ) ;
#17050=DIRECTION ( 'NONE',  ( 0.000000000000000000, 0.000000000000000000, 1.000000000000000000 ) ) ;
#17053=ORIENTED_EDGE ( 'NONE', *, *, #20100, .T. ) ;
#17055=ORIENTED_EDGE ( 'NONE', *, *, #13494, .T. ) ;
#17079=ORIENTED_EDGE ( 'NONE', *, *, #5251, .F. ) ;
#17125=EDGE_CURVE ( 'NONE', #9946, #6087, #248, .T. ) ;
#17126=CIRCLE ( 'NONE', #8618, 17.50000000000000355 ) ;
#17142=CIRCLE ( 'NONE', #8317, 7.500000000000020428 ) ;
#17152=VECTOR ( 'NONE', #4092, 1000.000000000000000 ) ;
#17163=VERTEX_POINT ( 'NONE', #17183 ) ;
#17178=DIRECTION ( 'NONE',  ( 0.7818314824680226982, 0.6234898018587423651, 0.000000000000000000 ) ) ;
#17183=CARTESIAN_POINT ( 'NONE',  ( 141.8714406926368099, -48.70825716237082759, 60.00000000000000000 ) ) ;
#17191=VERTEX_POINT ( 'NONE', #1524 ) ;
#17194=AXIS2_PLACEMENT_3D ( 'NONE', #17873, #19593, #778 ) ;
#17200=CIRCLE ( 'NONE', #3146, 7.500000000000020428 ) ;
#17210=AXIS2_PLACEMENT_3D ( 'NONE', #19762, #10252, #1142 ) ;
#17243=EDGE_CURVE ( 'NONE', #17330, #8799, #17896, .T. ) ;
#17257=CIRCLE ( 'NONE', #10363, 7.500000000000007105 ) ;
#17270=ADVANCED_FACE ( 'NONE', ( #14310 ), #187, .T. ) ;
#17272=FACE_BOUND ( 'NONE', #13043, .T. ) ;
#17273=AXIS2_PLACEMENT_3D ( 'NONE', #6770, #3493, #3595 ) ;
#17294=EDGE_LOOP ( 'NONE', ( #7288, #4666, #5408, #18007 ) ) ;
#17297=ORIENTED_EDGE ( 'NONE', *, *, #10465, .T. ) ;
#17298=EDGE_CURVE ( 'NONE', #17394, #16556, #12657, .T. ) ;
#17305=CIRCLE ( 'NONE', #19891, 150.0000000000000284 ) ;
#17308=EDGE_CURVE ( 'NONE', #625, #10243, #11437, .T. ) ;
#17330=VERTEX_POINT ( 'NONE', #2035 ) ;
#17350=ORIENTED_EDGE ( 'NONE', *, *, #9242, .F. ) ;
#17355=CARTESIAN_POINT ( 'NONE',  ( -159.9599531637108782, -36.50981547337168109, 60.00000000000000000 ) ) ;
#17379=CARTESIAN_POINT ( 'NONE',  ( -71.18887634719365565, -147.8252249328922687, 60.00000000000000000 ) ) ;
#17390=DIRECTION ( 'NONE',  ( -0.000000000000000000, -0.000000000000000000, -1.000000000000000000 ) ) ;
#17394=VERTEX_POINT ( 'NONE', #19419 ) ;
#17451=ORIENTED_EDGE ( 'NONE', *, *, #17779, .F. ) ;
#17466=DIRECTION ( 'NONE',  ( 1.000000000000000000, 0.000000000000000000, 0.000000000000000000 ) ) ;
#17477=CARTESIAN_POINT ( 'NONE',  ( -56.84754764479025368, -154.7316448359455308, 60.00000000000000000 ) ) ;
#17482=CARTESIAN_POINT ( 'NONE',  ( 138.2024300533213932, 89.85329105948596862, 60.00000000000000000 ) ) ;
#17484=FACE_OUTER_BOUND ( 'NONE', #13886, .T. ) ;
#17489=DIRECTION ( 'NONE',  ( 0.000000000000000000, 0.000000000000000000, 1.000000000000000000 ) ) ;
#17511=CARTESIAN_POINT ( 'NONE',  ( 159.9599531637113330, -36.50981547336952104, 60.00000000000000000 ) ) ;
#17524=VERTEX_POINT ( 'NONE', #7425 ) ;
#17547=EDGE_CURVE ( 'NONE', #16612, #698, #2540, .T. ) ;
#17569=ORIENTED_EDGE ( 'NONE', *, *, #17746, .T. ) ;
#17570=AXIS2_PLACEMENT_3D ( 'NONE', #18503, #18611, #10507 ) ;
#17571=ORIENTED_EDGE ( 'NONE', *, *, #5282, .F. ) ;
#17596=ORIENTED_EDGE ( 'NONE', *, *, #6285, .F. ) ;
#17597=DIRECTION ( 'NONE',  ( 0.000000000000000000, 0.000000000000000000, 1.000000000000000000 ) ) ;
#17601=FACE_BOUND ( 'NONE', #11346, .T. ) ;
#17602=EDGE_LOOP ( 'NONE', ( #5908, #4122, #8399, #2986 ) ) ;
#17625=EDGE_LOOP ( 'NONE', ( #8444, #19447, #8427, #10618 ) ) ;
#17639=CARTESIAN_POINT ( 'NONE',  ( 128.2779226595531270, 102.2982297021113141, 49.99999999999999289 ) ) ;
#17651=ORIENTED_EDGE ( 'NONE', *, *, #262, .F. ) ;
#17655=EDGE_CURVE ( 'NONE', #17163, #17877, #13504, .T. ) ;
#17660=CYLINDRICAL_SURFACE ( 'NONE', #13669, 15.91767397667354089 ) ;
#17700=VERTEX_POINT ( 'NONE', #5452 ) ;
#17712=CARTESIAN_POINT ( 'NONE',  ( -159.9599531637108782, -36.50981547337168109, 60.00000000000000000 ) ) ;
#17716=EDGE_LOOP ( 'NONE', ( #11586, #711, #11472, #18800 ) ) ;
#17722=SHAPE_DEFINITION_REPRESENTATION ( #7837, #7558 ) ;
#17732=CARTESIAN_POINT ( 'NONE',  ( 126.5370453525553671, 80.55045718954892209, 60.00000000000000000 ) ) ;
#17746=EDGE_CURVE ( 'NONE', #1319, #11007, #17257, .T. ) ;
#17749=AXIS2_PLACEMENT_3D ( 'NONE', #14140, #10760, #18858 ) ;
#17770=CARTESIAN_POINT ( 'NONE',  ( 71.18887634719571622, -147.8252249328912740, 49.99999999999999289 ) ) ;
#17779=EDGE_CURVE ( 'NONE', #14411, #9076, #893, .T. ) ;
#17790=CARTESIAN_POINT ( 'NONE',  ( -152.4599531637108498, -36.50981547337168109, 60.00000000000000000 ) ) ;
#17803=EDGE_LOOP ( 'NONE', ( #10091, #7968 ) ) ;
#17815=VERTEX_POINT ( 'NONE', #2988 ) ;
#17835=CARTESIAN_POINT ( 'NONE',  ( 50.37374754117451658, -141.2886604036503115, 49.99999999999999289 ) ) ;
#17867=CIRCLE ( 'NONE', #4444, 150.0000000000000284 ) ;
#17873=CARTESIAN_POINT ( 'NONE',  ( -71.18887634719365565, -147.8252249328922687, 60.00000000000000000 ) ) ;
#17877=VERTEX_POINT ( 'NONE', #10748 ) ;
#17896=CIRCLE ( 'NONE', #1552, 7.500000000000007105 ) ;
#17906=CYLINDRICAL_SURFACE ( 'NONE', #18780, 15.91767397667354089 ) ;
#17911=DIRECTION ( 'NONE',  ( -0.4338837391175662805, 0.9009688679024152602, 0.000000000000000000 ) ) ;
#17920=ADVANCED_FACE ( 'NONE', ( #212 ), #19252, .F. ) ;
#17944=AXIS2_PLACEMENT_3D ( 'NONE', #8281, #11740, #18002 ) ;
#17975=VERTEX_POINT ( 'NONE', #6367 ) ;
#17982=DIRECTION ( 'NONE',  ( 1.000000000000000000, 0.000000000000000000, 0.000000000000000000 ) ) ;
#18002=DIRECTION ( 'NONE',  ( 1.000000000000000000, 0.000000000000000000, 0.000000000000000000 ) ) ;
#18005=CARTESIAN_POINT ( 'NONE',  ( -159.9599531637108782, -36.50981547337168109, 49.99999999999999289 ) ) ;
#18006=AXIS2_PLACEMENT_3D ( 'NONE', #8356, #9794, #5005 ) ;
#18007=ORIENTED_EDGE ( 'NONE', *, *, #11610, .T. ) ;
#18031=DIRECTION ( 'NONE',  ( 0.000000000000000000, 0.000000000000000000, 1.000000000000000000 ) ) ;
#18038=EDGE_CURVE ( 'NONE', #17975, #6230, #10078, .T. ) ;
#18105=CARTESIAN_POINT ( 'NONE',  ( -148.9554720520392834, -17.67108784863415138, 49.99999999999999289 ) ) ;
#18109=EDGE_CURVE ( 'NONE', #3934, #14411, #14732, .T. ) ;
#18129=ORIENTED_EDGE ( 'NONE', *, *, #16410, .T. ) ;
#18131=( LENGTH_UNIT ( ) NAMED_UNIT ( * ) SI_UNIT ( .MILLI., .METRE. ) );
#18136=EDGE_LOOP ( 'NONE', ( #11798, #12667, #19912, #12702 ) ) ;
#18144=DIRECTION ( 'NONE',  ( 1.000000000000000000, 0.000000000000000000, 0.000000000000000000 ) ) ;
#18150=DIRECTION ( 'NONE',  ( -0.7818314824680222541, -0.6234898018587428092, 0.000000000000000000 ) ) ;
#18153=ORIENTED_EDGE ( 'NONE', *, *, #9531, .T. ) ;
#18177=CIRCLE ( 'NONE', #1181, 7.500000000000020428 ) ;
#18192=AXIS2_PLACEMENT_3D ( 'NONE', #7569, #1445, #15455 ) ;
#18199=FACE_OUTER_BOUND ( 'NONE', #18136, .T. ) ;
#18231=EDGE_CURVE ( 'NONE', #14483, #18743, #12358, .T. ) ;
#18232=AXIS2_PLACEMENT_3D ( 'NONE', #16869, #16673, #8882 ) ;
#18251=ADVANCED_FACE ( 'NONE', ( #2660 ), #15127, .F. ) ;
#18263=CARTESIAN_POINT ( 'NONE',  ( 167.4599531637113330, -36.50981547336952104, 60.00000000000000000 ) ) ;
#18279=DIRECTION ( 'NONE',  ( 1.000000000000000000, 0.000000000000000000, 0.000000000000000000 ) ) ;
#18282=ORIENTED_EDGE ( 'NONE', *, *, #2525, .F. ) ;
#18296=LINE ( 'NONE', #1092, #19760 ) ;
#18332=DIRECTION ( 'NONE',  ( -0.000000000000000000, -0.000000000000000000, -1.000000000000000000 ) ) ;
#18346=ORIENTED_EDGE ( 'NONE', *, *, #5987, .T. ) ;
#18354=ORIENTED_EDGE ( 'NONE', *, *, #258, .T. ) ;
#18371=ORIENTED_EDGE ( 'NONE', *, *, #7785, .T. ) ;
#18399=ORIENTED_EDGE ( 'NONE', *, *, #1740, .F. ) ;
#18412=DIRECTION ( 'NONE',  ( 1.000000000000000000, 0.000000000000000000, 0.000000000000000000 ) ) ;
#18458=ORIENTED_EDGE ( 'NONE', *, *, #17298, .T. ) ;
#18490=CARTESIAN_POINT ( 'NONE',  ( -7.500000000000008882, 164.0736214083062805, 60.00000000000000000 ) ) ;
#18501=VECTOR ( 'NONE', #13554, 1000.000000000000000 ) ;
#18503=CARTESIAN_POINT ( 'NONE',  ( -71.18887634719365565, -147.8252249328922687, 49.99999999999999289 ) ) ;
#18516=LINE ( 'NONE', #6251, #2936 ) ;
#18520=ORIENTED_EDGE ( 'NONE', *, *, #2630, .F. ) ;
#18539=ORIENTED_EDGE ( 'NONE', *, *, #8477, .F. ) ;
#18540=EDGE_CURVE ( 'NONE', #9011, #4491, #5197, .T. ) ;
#18546=LINE ( 'NONE', #9018, #4166 ) ;
#18547=CIRCLE ( 'NONE', #19844, 7.500000000000008882 ) ;
#18548=ADVANCED_FACE ( 'NONE', ( #18889 ), #17660, .T. ) ;
#18550=DIRECTION ( 'NONE',  ( -0.000000000000000000, -0.000000000000000000, -1.000000000000000000 ) ) ;
#18551=CARTESIAN_POINT ( 'NONE',  ( -156.4179374840092862, -52.02840013024096066, 60.00000000000000000 ) ) ;
#18563=AXIS2_PLACEMENT_3D ( 'NONE', #18784, #8024, #9566 ) ;
#18589=ORIENTED_EDGE ( 'NONE', *, *, #10789, .F. ) ;
#18599=EDGE_CURVE ( 'NONE', #13002, #6462, #15649, .T. ) ;
#18604=AXIS2_PLACEMENT_3D ( 'NONE', #5645, #19751, #16498 ) ;
#18611=DIRECTION ( 'NONE',  ( 0.000000000000000000, 0.000000000000000000, 1.000000000000000000 ) ) ;
#18618=DIRECTION ( 'NONE',  ( 0.000000000000000000, 0.000000000000000000, 1.000000000000000000 ) ) ;
#18639=AXIS2_PLACEMENT_3D ( 'NONE', #8416, #18031, #13500 ) ;
#18675=CIRCLE ( 'NONE', #3639, 7.500000000000007105 ) ;
#18694=CARTESIAN_POINT ( 'NONE',  ( 71.18887634719571622, -147.8252249328912740, 60.00000000000000000 ) ) ;
#18700=AXIS2_PLACEMENT_3D ( 'NONE', #17639, #39, #14049 ) ;
#18703=PLANE ( 'NONE',  #11060 ) ;
#18706=ORIENTED_EDGE ( 'NONE', *, *, #12400, .F. ) ;
#18707=CARTESIAN_POINT ( 'NONE',  ( 85.53020504959901871, -140.9188050298377846, 60.00000000000000000 ) ) ;
#18721=VERTEX_POINT ( 'NONE', #14963 ) ;
#18738=DIRECTION ( 'NONE',  ( -0.000000000000000000, -0.000000000000000000, -1.000000000000000000 ) ) ;
#18743=VERTEX_POINT ( 'NONE', #9968 ) ;
#18769=CARTESIAN_POINT ( 'NONE',  ( -79.05640494597940915, -127.4758205975444270, 60.00000000000000000 ) ) ;
#18775=ADVANCED_FACE ( 'NONE', ( #10768 ), #16711, .F. ) ;
#18780=AXIS2_PLACEMENT_3D ( 'NONE', #19338, #5323, #5719 ) ;
#18784=CARTESIAN_POINT ( 'NONE',  ( 159.9599531637113330, -36.50981547336952104, 49.99999999999999289 ) ) ;
#18800=ORIENTED_EDGE ( 'NONE', *, *, #3855, .T. ) ;
#18801=EDGE_CURVE ( 'NONE', #12677, #10504, #1363, .T. ) ;
#18818=DIRECTION ( 'NONE',  ( 1.000000000000000000, 0.000000000000000000, 0.000000000000000000 ) ) ;
#18826=CYLINDRICAL_SURFACE ( 'NONE', #14485, 7.500000000000020428 ) ;
#18827=ORIENTED_EDGE ( 'NONE', *, *, #12108, .T. ) ;
#18858=DIRECTION ( 'NONE',  ( 1.000000000000000000, 0.000000000000000000, 0.000000000000000000 ) ) ;
#18880=AXIS2_PLACEMENT_3D ( 'NONE', #10994, #3233, #1697 ) ;
#18889=FACE_OUTER_BOUND ( 'NONE', #7729, .T. ) ;
#18900=ORIENTED_EDGE ( 'NONE', *, *, #16412, .F. ) ;
#18909=LINE ( 'NONE', #14087, #3223 ) ;
#18920=DIRECTION ( 'NONE',  ( 0.9749279121818223981, 0.2225209339563194444, 0.000000000000000000 ) ) ;
#18927=VECTOR ( 'NONE', #19869, 1000.000000000000227 ) ;
#18974=DIRECTION ( 'NONE',  ( 0.000000000000000000, 0.000000000000000000, 1.000000000000000000 ) ) ;
#19000=DIRECTION ( 'NONE',  ( 0.000000000000000000, 0.000000000000000000, 1.000000000000000000 ) ) ;
#19017=CARTESIAN_POINT ( 'NONE',  ( -15.91767397667354800, 164.0736214083062805, 60.00000000000000000 ) ) ;
#19021=DIRECTION ( 'NONE',  ( -1.000000000000000000, 0.000000000000000000, 0.000000000000000000 ) ) ;
#19045=VECTOR ( 'NONE', #5446, 1000.000000000000000 ) ;
#19053=DIRECTION ( 'NONE',  ( 1.000000000000000000, 0.000000000000000000, 0.000000000000000000 ) ) ;
#19075=VECTOR ( 'NONE', #12703, 1000.000000000000000 ) ;
#19076=DIRECTION ( 'NONE',  ( -1.000000000000000000, 0.000000000000000000, 0.000000000000000000 ) ) ;
#19090=DIRECTION ( 'NONE',  ( 1.000000000000000000, 0.000000000000000000, 0.000000000000000000 ) ) ;
#19102=ORIENTED_EDGE ( 'NONE', *, *, #17243, .T. ) ;
#19120=CARTESIAN_POINT ( 'NONE',  ( -56.84754764479025368, -154.7316448359455308, 60.00000000000000000 ) ) ;
#19133=ORIENTED_EDGE ( 'NONE', *, *, #8735, .F. ) ;
#19170=DIRECTION ( 'NONE',  ( -1.000000000000000000, 0.000000000000000000, 0.000000000000000000 ) ) ;
#19178=ORIENTED_EDGE ( 'NONE', *, *, #2630, .T. ) ;
#19219=EDGE_CURVE ( 'NONE', #8799, #17330, #9809, .T. ) ;
#19222=CARTESIAN_POINT ( 'NONE',  ( -148.9554720520392834, -17.67108784863415138, 49.99999999999999289 ) ) ;
#19229=DIRECTION ( 'NONE',  ( -0.000000000000000000, -0.000000000000000000, -1.000000000000000000 ) ) ;
#19234=PLANE ( 'NONE',  #10546 ) ;
#19237=CARTESIAN_POINT ( 'NONE',  ( 118.3534152657848608, 114.7431683447366595, 60.00000000000000000 ) ) ;
#19243=CARTESIAN_POINT ( 'NONE',  ( 0.000000000000000000, 0.000000000000000000, 60.00000000000000000 ) ) ;
#19252=PLANE ( 'NONE',  #17273 ) ;
#19256=ORIENTED_EDGE ( 'NONE', *, *, #15498, .T. ) ;
#19285=ORIENTED_EDGE ( 'NONE', *, *, #19219, .F. ) ;
#19287=CARTESIAN_POINT ( 'NONE',  ( 63.68887634719569490, -147.8252249328912740, 49.99999999999999289 ) ) ;
#19295=LINE ( 'NONE', #8134, #8087 ) ;
#19301=ORIENTED_EDGE ( 'NONE', *, *, #19446, .T. ) ;
#19306=ORIENTED_EDGE ( 'NONE', *, *, #1740, .T. ) ;
#19312=AXIS2_PLACEMENT_3D ( 'NONE', #2257, #8486, #2058 ) ;
#19318=CARTESIAN_POINT ( 'NONE',  ( -71.18887634719365565, -147.8252249328922687, 60.00000000000000000 ) ) ;
#19324=CARTESIAN_POINT ( 'NONE',  ( 0.000000000000000000, 0.000000000000000000, 60.00000000000000000 ) ) ;
#19329=VERTEX_POINT ( 'NONE', #12982 ) ;
#19338=CARTESIAN_POINT ( 'NONE',  ( -159.9599531637108782, -36.50981547337168109, 60.00000000000000000 ) ) ;
#19346=DIRECTION ( 'NONE',  ( 1.000000000000000000, 0.000000000000000000, 0.000000000000000000 ) ) ;
#19347=EDGE_LOOP ( 'NONE', ( #15716, #11847, #15535, #9286 ) ) ;
#19393=EDGE_CURVE ( 'NONE', #1887, #15200, #11741, .T. ) ;
#19413=LINE ( 'NONE', #2330, #3568 ) ;
#19415=EDGE_CURVE ( 'NONE', #10, #17163, #6571, .T. ) ;
#19419=CARTESIAN_POINT ( 'NONE',  ( 138.2024300533213932, 89.85329105948596862, 60.00000000000000000 ) ) ;
#19425=CARTESIAN_POINT ( 'NONE',  ( -15.91767397667355510, 149.1530343478547422, 49.99999999999999289 ) ) ;
#19433=STYLED_ITEM ( 'NONE', ( #4300 ), #14854 ) ;
#19445=DIRECTION ( 'NONE',  ( -1.000000000000000000, 0.000000000000000000, 0.000000000000000000 ) ) ;
#19446=EDGE_CURVE ( 'NONE', #12253, #6115, #3308, .T. ) ;
#19447=ORIENTED_EDGE ( 'NONE', *, *, #7977, .T. ) ;
#19463=LINE ( 'NONE', #19554, #19045 ) ;
#19484=DIRECTION ( 'NONE',  ( 0.000000000000000000, 0.000000000000000000, 1.000000000000000000 ) ) ;
#19485=LINE ( 'NONE', #760, #13297 ) ;
#19488=VECTOR ( 'NONE', #17178, 1000.000000000000114 ) ;
#19489=ORIENTED_EDGE ( 'NONE', *, *, #19393, .T. ) ;
#19523=DIRECTION ( 'NONE',  ( 1.000000000000000000, 0.000000000000000000, 0.000000000000000000 ) ) ;
#19528=LINE ( 'NONE', #16272, #12699 ) ;
#19539=AXIS2_PLACEMENT_3D ( 'NONE', #15459, #3192, #19955 ) ;
#19554=CARTESIAN_POINT ( 'NONE',  ( 63.68887634719569490, -147.8252249328912740, 60.00000000000000000 ) ) ;
#19556=CARTESIAN_POINT ( 'NONE',  ( 71.18887634719571622, -147.8252249328912740, 60.00000000000000000 ) ) ;
#19560=LINE ( 'NONE', #7190, #2367 ) ;
#19565=LINE ( 'NONE', #5557, #6090 ) ;
#19582=ORIENTED_EDGE ( 'NONE', *, *, #7705, .F. ) ;
#19593=DIRECTION ( 'NONE',  ( 0.000000000000000000, 0.000000000000000000, 1.000000000000000000 ) ) ;
#19602=DIRECTION ( 'NONE',  ( -1.000000000000000000, 0.000000000000000000, 0.000000000000000000 ) ) ;
#19604=EDGE_CURVE ( 'NONE', #625, #12873, #15045, .T. ) ;
#19605=DIRECTION ( 'NONE',  ( 1.000000000000000000, 0.000000000000000000, 0.000000000000000000 ) ) ;
#19619=DIRECTION ( 'NONE',  ( 0.000000000000000000, 0.000000000000000000, 1.000000000000000000 ) ) ;
#19633=ORIENTED_EDGE ( 'NONE', *, *, #4544, .T. ) ;
#19636=FACE_OUTER_BOUND ( 'NONE', #1890, .T. ) ;
#19641=LINE ( 'NONE', #4191, #16645 ) ;
#19665=CARTESIAN_POINT ( 'NONE',  ( 79.05640494598117129, -127.4758205975433327, 60.00000000000000000 ) ) ;
#19682=ORIENTED_EDGE ( 'NONE', *, *, #10622, .T. ) ;
#19715=CYLINDRICAL_SURFACE ( 'NONE', #10281, 7.500000000000007105 ) ;
#19732=ORIENTED_EDGE ( 'NONE', *, *, #8415, .T. ) ;
#19744=CARTESIAN_POINT ( 'NONE',  ( 167.4599531637113330, -36.50981547336952104, 60.00000000000000000 ) ) ;
#19751=DIRECTION ( 'NONE',  ( -0.000000000000000000, -0.000000000000000000, -1.000000000000000000 ) ) ;
#19755=DIRECTION ( 'NONE',  ( 0.9749279121818261729, -0.2225209339563031519, 0.000000000000000000 ) ) ;
#19760=VECTOR ( 'NONE', #19818, 1000.000000000000000 ) ;
#19762=CARTESIAN_POINT ( 'NONE',  ( 0.000000000000000000, 0.000000000000000000, 49.99999999999999289 ) ) ;
#19780=ADVANCED_FACE ( 'NONE', ( #14870 ), #10073, .F. ) ;
#19786=ORIENTED_EDGE ( 'NONE', *, *, #19415, .F. ) ;
#19792=EDGE_LOOP ( 'NONE', ( #12823, #8711, #19133, #4367 ) ) ;
#19800=CYLINDRICAL_SURFACE ( 'NONE', #12439, 15.91767397667355510 ) ;
#19818=DIRECTION ( 'NONE',  ( -0.000000000000000000, -0.000000000000000000, -1.000000000000000000 ) ) ;
#19835=CIRCLE ( 'NONE', #18880, 7.500000000000007105 ) ;
#19843=EDGE_CURVE ( 'NONE', #16987, #6676, #4283, .T. ) ;
#19844=AXIS2_PLACEMENT_3D ( 'NONE', #1711, #3452, #4901 ) ;
#19865=DIRECTION ( 'NONE',  ( -0.000000000000000000, -0.000000000000000000, -1.000000000000000000 ) ) ;
#19869=DIRECTION ( 'NONE',  ( 0.4338837391175549563, 0.9009688679024205893, 0.000000000000000000 ) ) ;
#19877=FACE_OUTER_BOUND ( 'NONE', #8960, .T. ) ;
#19883=LINE ( 'NONE', #4235, #10196 ) ;
#19891=AXIS2_PLACEMENT_3D ( 'NONE', #12861, #13149, #5300 ) ;
#19912=ORIENTED_EDGE ( 'NONE', *, *, #7890, .F. ) ;
#19924=CARTESIAN_POINT ( 'NONE',  ( 0.000000000000000000, 164.0736214083062805, 60.00000000000000000 ) ) ;
#19930=DIRECTION ( 'NONE',  ( -4.650550193362991910E-16, -1.000000000000000000, 0.000000000000000000 ) ) ;
#19940=ORIENTED_EDGE ( 'NONE', *, *, #987, .F. ) ;
#19955=DIRECTION ( 'NONE',  ( 1.000000000000000000, 0.000000000000000000, 0.000000000000000000 ) ) ;
#20000=LINE ( 'NONE', #2429, #14346 ) ;
#20005=CARTESIAN_POINT ( 'NONE',  ( -17.49999999999999289, 0.000000000000000000, 49.99999999999999289 ) ) ;
#20009=DIRECTION ( 'NONE',  ( -4.650550193362991910E-16, -1.000000000000000000, 0.000000000000000000 ) ) ;
#20010=AXIS2_PLACEMENT_3D ( 'NONE', #2359, #4082, #19346 ) ;
#20015=ORIENTED_EDGE ( 'NONE', *, *, #16413, .F. ) ;
#20020=DIRECTION ( 'NONE',  ( -0.000000000000000000, -0.000000000000000000, -1.000000000000000000 ) ) ;
#20028=EDGE_CURVE ( 'NONE', #12028, #6717, #2007, .T. ) ;
#20039=DIRECTION ( 'NONE',  ( -0.000000000000000000, -0.000000000000000000, -1.000000000000000000 ) ) ;
#20041=ORIENTED_EDGE ( 'NONE', *, *, #7977, .F. ) ;
#20043=EDGE_LOOP ( 'NONE', ( #11683, #6943, #1385, #3911 ) ) ;
#20045=VECTOR ( 'NONE', #3760, 1000.000000000000000 ) ;
#20053=ADVANCED_FACE ( 'NONE', ( #3617 ), #12608, .T. ) ;
#20070=ORIENTED_EDGE ( 'NONE', *, *, #15010, .F. ) ;
#20095=FACE_OUTER_BOUND ( 'NONE', #5790, .T. ) ;
#20100=EDGE_CURVE ( 'NONE', #12873, #625, #18675, .T. ) ;
#20112=VERTEX_POINT ( 'NONE', #8009 ) ;
#20117=EDGE_LOOP ( 'NONE', ( #14875, #1668 ) ) ;
#20125=CIRCLE ( 'NONE', #11312, 15.91767397667355510 ) ;
#20136=ORIENTED_EDGE ( 'NONE', *, *, #2673, .T. ) ;
#20157=( LENGTH_UNIT ( ) NAMED_UNIT ( * ) SI_UNIT ( .MILLI., .METRE. ) );
#20169=VERTEX_POINT ( 'NONE', #3906 ) ;
#20185=DIRECTION ( 'NONE',  ( -0.000000000000000000, -0.000000000000000000, -1.000000000000000000 ) ) ;
#20223=CARTESIAN_POINT ( 'NONE',  ( -85.53020504959707182, -140.9188050298390067, 60.00000000000000000 ) ) ;
#20224=FACE_BOUND ( 'NONE', #15129, .T. ) ;
#20228=FACE_OUTER_BOUND ( 'NONE', #17716, .T. ) ;
ENDSEC;
END-ISO-10303-21;
